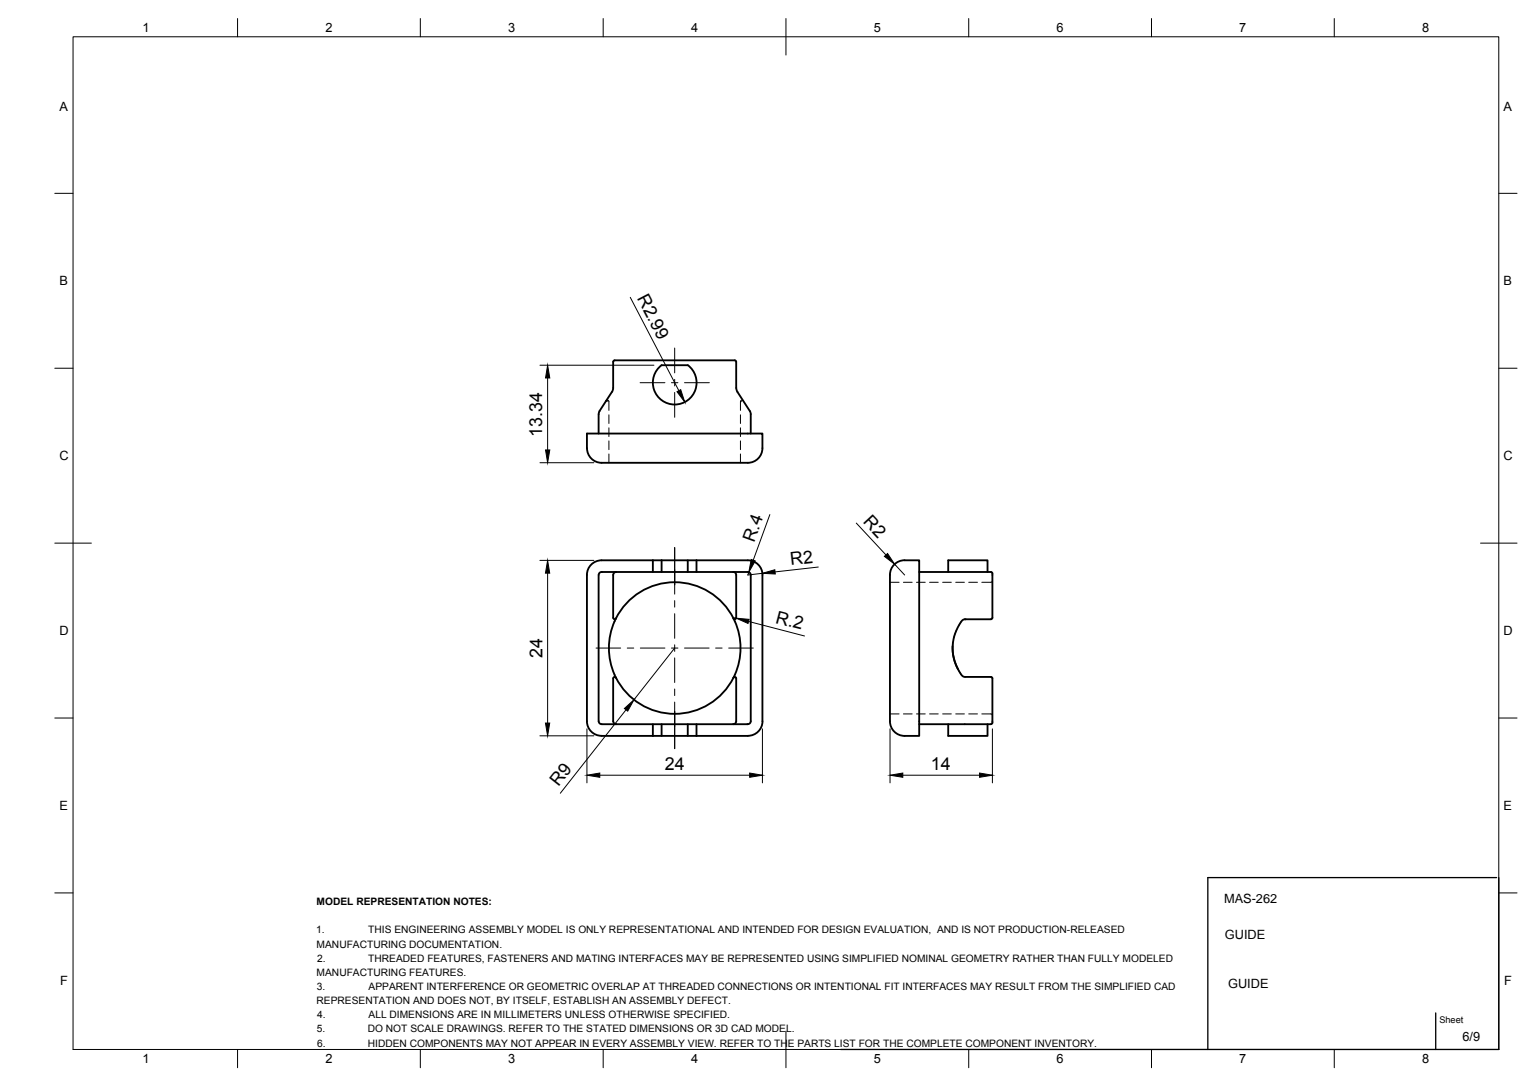
ISO-10303-21;
HEADER;
/* Generated by software containing ST-Developer
 * from STEP Tools, Inc. (www.steptools.com) 
 */

FILE_DESCRIPTION(
/* description */ (''),
/* implementation_level */ '2;1');

FILE_NAME(
/* name */ 'GUIDE.step',
/* time_stamp */ '2026-10-07T02:13:48+06:00',
/* author */ (''),
/* organization */ (''),
/* preprocessor_version */ 'ST-DEVELOPER v20.2',
/* originating_system */ 'Autodesk Translation Framework v15.15.0.0',
/* authorisation */ '');

FILE_SCHEMA (('AUTOMOTIVE_DESIGN { 1 0 10303 214 3 1 1 }'));
ENDSEC;

DATA;
#10=MECHANICAL_DESIGN_GEOMETRIC_PRESENTATION_REPRESENTATION('',(#117),#17042);
#70=B_SPLINE_SURFACE_WITH_KNOTS('',3,3,((#13032,#13033,#13034,#13035,#13036),
(#13037,#13038,#13039,#13040,#13041),(#13042,#13043,#13044,#13045,#13046),
(#13047,#13048,#13049,#13050,#13051),(#13052,#13053,#13054,#13055,#13056),
(#13057,#13058,#13059,#13060,#13061),(#13062,#13063,#13064,#13065,#13066)),
 .UNSPECIFIED.,.F.,.F.,.F.,(4,1,1,1,4),(4,1,4),(0.,0.285714285714286,0.571428571428571,
0.857142857142857,1.),(0.,0.020779022277979,0.0415580445559579),
 .UNSPECIFIED.);
#71=B_SPLINE_SURFACE_WITH_KNOTS('',3,3,((#13080,#13081,#13082,#13083,#13084,
#13085),(#13086,#13087,#13088,#13089,#13090,#13091),(#13092,#13093,#13094,
#13095,#13096,#13097),(#13098,#13099,#13100,#13101,#13102,#13103),(#13104,
#13105,#13106,#13107,#13108,#13109),(#13110,#13111,#13112,#13113,#13114,
#13115),(#13116,#13117,#13118,#13119,#13120,#13121)),.UNSPECIFIED.,.F.,
 .F.,.F.,(4,1,1,1,4),(4,1,1,4),(0.,0.285714285714286,0.571428571428571,
0.857142857142857,1.),(-0.417579612421967,-0.0596542303459957,0.178962691037985,
0.417579612421966),.UNSPECIFIED.);
#72=B_SPLINE_SURFACE_WITH_KNOTS('',3,3,((#13127,#13128,#13129,#13130,#13131),
(#13132,#13133,#13134,#13135,#13136),(#13137,#13138,#13139,#13140,#13141),
(#13142,#13143,#13144,#13145,#13146),(#13147,#13148,#13149,#13150,#13151),
(#13152,#13153,#13154,#13155,#13156),(#13157,#13158,#13159,#13160,#13161)),
 .UNSPECIFIED.,.F.,.F.,.F.,(4,1,1,1,4),(4,1,4),(0.,0.285714285714286,0.571428571428571,
0.857142857142857,1.),(0.,0.0207805027277528,0.0415610054555056),
 .UNSPECIFIED.);
#73=B_SPLINE_SURFACE_WITH_KNOTS('',3,3,((#13236,#13237,#13238,#13239,#13240),
(#13241,#13242,#13243,#13244,#13245),(#13246,#13247,#13248,#13249,#13250),
(#13251,#13252,#13253,#13254,#13255),(#13256,#13257,#13258,#13259,#13260),
(#13261,#13262,#13263,#13264,#13265),(#13266,#13267,#13268,#13269,#13270)),
 .UNSPECIFIED.,.F.,.F.,.F.,(4,1,1,1,4),(4,1,4),(0.,0.285714285714286,0.571428571428571,
0.857142857142857,1.),(0.,0.0207790222779789,0.0415580445559579),
 .UNSPECIFIED.);
#74=B_SPLINE_SURFACE_WITH_KNOTS('',3,3,((#13284,#13285,#13286,#13287,#13288,
#13289),(#13290,#13291,#13292,#13293,#13294,#13295),(#13296,#13297,#13298,
#13299,#13300,#13301),(#13302,#13303,#13304,#13305,#13306,#13307),(#13308,
#13309,#13310,#13311,#13312,#13313),(#13314,#13315,#13316,#13317,#13318,
#13319),(#13320,#13321,#13322,#13323,#13324,#13325)),.UNSPECIFIED.,.F.,
 .F.,.F.,(4,1,1,1,4),(4,1,1,4),(0.,0.285714285714286,0.571428571428571,
0.857142857142857,1.),(-0.417579612421968,-0.0596542303459959,0.178962691037985,
0.417579612421966),.UNSPECIFIED.);
#75=B_SPLINE_SURFACE_WITH_KNOTS('',3,3,((#13331,#13332,#13333,#13334,#13335),
(#13336,#13337,#13338,#13339,#13340),(#13341,#13342,#13343,#13344,#13345),
(#13346,#13347,#13348,#13349,#13350),(#13351,#13352,#13353,#13354,#13355),
(#13356,#13357,#13358,#13359,#13360),(#13361,#13362,#13363,#13364,#13365)),
 .UNSPECIFIED.,.F.,.F.,.F.,(4,1,1,1,4),(4,1,4),(0.,0.285714285714286,0.571428571428571,
0.857142857142857,1.),(0.,0.0207805027277526,0.0415610054555052),
 .UNSPECIFIED.);
#93=SHAPE_REPRESENTATION_RELATIONSHIP('SRR','None',#17089,#105);
#105=ADVANCED_BREP_SHAPE_REPRESENTATION('',(#129),#17033);
#117=STYLED_ITEM('',(#17154),#129);
#129=MANIFOLD_SOLID_BREP('Body1',#8118);
#158=FACE_BOUND('',#1181,.T.);
#159=FACE_BOUND('',#1228,.T.);
#160=FACE_BOUND('',#1237,.T.);
#161=FACE_BOUND('',#1260,.T.);
#188=(
BOUNDED_SURFACE()
B_SPLINE_SURFACE(2,2,((#13423,#13424,#13425),(#13426,#13427,#13428),(#13429,
#13430,#13431)),.UNSPECIFIED.,.F.,.F.,.F.)
B_SPLINE_SURFACE_WITH_KNOTS((3,3),(3,3),(-1.5707963267949,1.77635683940025E-13),
(0.,1.5707963267949),.UNSPECIFIED.)
GEOMETRIC_REPRESENTATION_ITEM()
RATIONAL_B_SPLINE_SURFACE(((1.,0.707106781186548,1.),(0.707106781186393,
0.499999999999891,0.707106781186393),(1.,0.707106781186548,1.)))
REPRESENTATION_ITEM('')
SURFACE()
);
#189=(
BOUNDED_SURFACE()
B_SPLINE_SURFACE(2,2,((#13443,#13444,#13445),(#13446,#13447,#13448),(#13449,
#13450,#13451)),.UNSPECIFIED.,.F.,.F.,.F.)
B_SPLINE_SURFACE_WITH_KNOTS((3,3),(3,3),(-1.5707963267949,0.),(-1.5707963267949,
5.55111512312578E-15),.UNSPECIFIED.)
GEOMETRIC_REPRESENTATION_ITEM()
RATIONAL_B_SPLINE_SURFACE(((1.,0.707106781186546,1.),(0.707106781186793,
0.500000000000172,0.707106781186793),(1.,0.707106781186546,1.)))
REPRESENTATION_ITEM('')
SURFACE()
);
#190=(
BOUNDED_SURFACE()
B_SPLINE_SURFACE(2,2,((#13465,#13466,#13467),(#13468,#13469,#13470),(#13471,
#13472,#13473)),.UNSPECIFIED.,.F.,.F.,.F.)
B_SPLINE_SURFACE_WITH_KNOTS((3,3),(3,3),(-1.5707963267949,0.),(-3.14159265358979,
-1.5707963267949),.UNSPECIFIED.)
GEOMETRIC_REPRESENTATION_ITEM()
RATIONAL_B_SPLINE_SURFACE(((1.,0.707106781186548,1.),(0.707106781186801,
0.50000000000018,0.707106781186801),(1.,0.707106781186548,1.)))
REPRESENTATION_ITEM('')
SURFACE()
);
#191=(
BOUNDED_SURFACE()
B_SPLINE_SURFACE(2,2,((#13485,#13486,#13487),(#13488,#13489,#13490),(#13491,
#13492,#13493)),.UNSPECIFIED.,.F.,.F.,.F.)
B_SPLINE_SURFACE_WITH_KNOTS((3,3),(3,3),(-1.5707963267949,0.),(1.5707963267949,
3.14159265358979),.UNSPECIFIED.)
GEOMETRIC_REPRESENTATION_ITEM()
RATIONAL_B_SPLINE_SURFACE(((1.,0.707106781186547,1.),(0.707106781186801,
0.500000000000179,0.707106781186801),(1.,0.707106781186547,1.)))
REPRESENTATION_ITEM('')
SURFACE()
);
#192=(
BOUNDED_SURFACE()
B_SPLINE_SURFACE(2,2,((#13513,#13514,#13515),(#13516,#13517,#13518),(#13519,
#13520,#13521)),.UNSPECIFIED.,.F.,.F.,.F.)
B_SPLINE_SURFACE_WITH_KNOTS((3,3),(3,3),(-8.32667268468867E-15,1.57079632679493),
(-1.57079632679491,-0.994301061223377),.UNSPECIFIED.)
GEOMETRIC_REPRESENTATION_ITEM()
RATIONAL_B_SPLINE_SURFACE(((1.,0.958743497277462,1.),(0.707106781186526,
0.677934028343379,0.707106781186526),(1.,0.958743497277462,1.)))
REPRESENTATION_ITEM('')
SURFACE()
);
#193=(
BOUNDED_SURFACE()
B_SPLINE_SURFACE(2,2,((#13547,#13548,#13549),(#13550,#13551,#13552),(#13553,
#13554,#13555)),.UNSPECIFIED.,.F.,.F.,.F.)
B_SPLINE_SURFACE_WITH_KNOTS((3,3),(3,3),(0.,1.57079632679491),(0.994301061223376,
1.5707963267949),.UNSPECIFIED.)
GEOMETRIC_REPRESENTATION_ITEM()
RATIONAL_B_SPLINE_SURFACE(((1.,0.958743497277463,1.),(0.707106781186533,
0.677934028343387,0.707106781186533),(1.,0.958743497277463,1.)))
REPRESENTATION_ITEM('')
SURFACE()
);
#194=(
BOUNDED_SURFACE()
B_SPLINE_SURFACE(2,2,((#13571,#13572,#13573),(#13574,#13575,#13576),(#13577,
#13578,#13579)),.UNSPECIFIED.,.F.,.F.,.F.)
B_SPLINE_SURFACE_WITH_KNOTS((3,3),(3,3),(0.,1.57079632679492),(1.5707963267949,
2.14729159236641),.UNSPECIFIED.)
GEOMETRIC_REPRESENTATION_ITEM()
RATIONAL_B_SPLINE_SURFACE(((1.,0.958743497277464,1.),(0.707106781186532,
0.677934028343386,0.707106781186532),(1.,0.958743497277464,1.)))
REPRESENTATION_ITEM('')
SURFACE()
);
#195=(
BOUNDED_SURFACE()
B_SPLINE_SURFACE(2,2,((#13605,#13606,#13607),(#13608,#13609,#13610),(#13611,
#13612,#13613)),.UNSPECIFIED.,.F.,.F.,.F.)
B_SPLINE_SURFACE_WITH_KNOTS((3,3),(3,3),(0.,1.57079632679492),(-2.14729159236642,
-1.57079632679489),.UNSPECIFIED.)
GEOMETRIC_REPRESENTATION_ITEM()
RATIONAL_B_SPLINE_SURFACE(((1.,0.958743497277463,1.),(0.707106781186532,
0.677934028343385,0.707106781186532),(1.,0.958743497277463,1.)))
REPRESENTATION_ITEM('')
SURFACE()
);
#202=SPHERICAL_SURFACE('',#8655,2.);
#203=SPHERICAL_SURFACE('',#8660,2.);
#204=SPHERICAL_SURFACE('',#8665,2.);
#205=SPHERICAL_SURFACE('',#8667,2.);
#206=SPHERICAL_SURFACE('',#8677,0.2);
#207=SPHERICAL_SURFACE('',#8690,0.2);
#208=SPHERICAL_SURFACE('',#8707,0.2);
#209=SPHERICAL_SURFACE('',#8720,0.2);
#220=TOROIDAL_SURFACE('',#8702,9.2,0.2);
#221=TOROIDAL_SURFACE('',#8731,9.2,0.2);
#222=TOROIDAL_SURFACE('',#8762,1.39999999999987,0.4);
#223=TOROIDAL_SURFACE('',#8773,1.39999999999987,0.4);
#224=TOROIDAL_SURFACE('',#8782,1.39999999999987,0.4);
#225=TOROIDAL_SURFACE('',#8793,1.39999999999987,0.4);
#240=ELLIPSE('',#8685,16.7697982864697,9.);
#241=ELLIPSE('',#8686,16.8779777985659,9.2);
#242=ELLIPSE('',#8715,16.7697982864697,9.);
#243=ELLIPSE('',#8716,16.8779777985659,9.2);
#370=PLANE('',#8671);
#371=PLANE('',#8674);
#372=PLANE('',#8675);
#373=PLANE('',#8693);
#374=PLANE('',#8696);
#375=PLANE('',#8699);
#376=PLANE('',#8722);
#377=PLANE('',#8725);
#378=PLANE('',#8728);
#379=PLANE('',#8746);
#380=PLANE('',#8758);
#381=PLANE('',#8769);
#382=PLANE('',#8789);
#383=PLANE('',#8801);
#384=PLANE('',#8802);
#385=PLANE('',#8805);
#386=PLANE('',#8806);
#387=PLANE('',#8807);
#388=PLANE('',#8808);
#389=PLANE('',#8821);
#390=PLANE('',#8824);
#391=PLANE('',#8825);
#671=FACE_OUTER_BOUND('',#1168,.T.);
#672=FACE_OUTER_BOUND('',#1169,.T.);
#673=FACE_OUTER_BOUND('',#1170,.T.);
#674=FACE_OUTER_BOUND('',#1171,.T.);
#675=FACE_OUTER_BOUND('',#1172,.T.);
#676=FACE_OUTER_BOUND('',#1173,.T.);
#677=FACE_OUTER_BOUND('',#1174,.T.);
#678=FACE_OUTER_BOUND('',#1175,.T.);
#679=FACE_OUTER_BOUND('',#1176,.T.);
#680=FACE_OUTER_BOUND('',#1177,.T.);
#681=FACE_OUTER_BOUND('',#1178,.T.);
#682=FACE_OUTER_BOUND('',#1179,.T.);
#683=FACE_OUTER_BOUND('',#1180,.T.);
#684=FACE_OUTER_BOUND('',#1182,.T.);
#685=FACE_OUTER_BOUND('',#1183,.T.);
#686=FACE_OUTER_BOUND('',#1184,.T.);
#687=FACE_OUTER_BOUND('',#1185,.T.);
#688=FACE_OUTER_BOUND('',#1186,.T.);
#689=FACE_OUTER_BOUND('',#1187,.T.);
#690=FACE_OUTER_BOUND('',#1188,.T.);
#691=FACE_OUTER_BOUND('',#1189,.T.);
#692=FACE_OUTER_BOUND('',#1190,.T.);
#693=FACE_OUTER_BOUND('',#1191,.T.);
#694=FACE_OUTER_BOUND('',#1192,.T.);
#695=FACE_OUTER_BOUND('',#1193,.T.);
#696=FACE_OUTER_BOUND('',#1194,.T.);
#697=FACE_OUTER_BOUND('',#1195,.T.);
#698=FACE_OUTER_BOUND('',#1196,.T.);
#699=FACE_OUTER_BOUND('',#1197,.T.);
#700=FACE_OUTER_BOUND('',#1198,.T.);
#701=FACE_OUTER_BOUND('',#1199,.T.);
#702=FACE_OUTER_BOUND('',#1200,.T.);
#703=FACE_OUTER_BOUND('',#1201,.T.);
#704=FACE_OUTER_BOUND('',#1202,.T.);
#705=FACE_OUTER_BOUND('',#1203,.T.);
#706=FACE_OUTER_BOUND('',#1204,.T.);
#707=FACE_OUTER_BOUND('',#1205,.T.);
#708=FACE_OUTER_BOUND('',#1206,.T.);
#709=FACE_OUTER_BOUND('',#1207,.T.);
#710=FACE_OUTER_BOUND('',#1208,.T.);
#711=FACE_OUTER_BOUND('',#1209,.T.);
#712=FACE_OUTER_BOUND('',#1210,.T.);
#713=FACE_OUTER_BOUND('',#1211,.T.);
#714=FACE_OUTER_BOUND('',#1212,.T.);
#715=FACE_OUTER_BOUND('',#1213,.T.);
#716=FACE_OUTER_BOUND('',#1214,.T.);
#717=FACE_OUTER_BOUND('',#1215,.T.);
#718=FACE_OUTER_BOUND('',#1216,.T.);
#719=FACE_OUTER_BOUND('',#1217,.T.);
#720=FACE_OUTER_BOUND('',#1218,.T.);
#721=FACE_OUTER_BOUND('',#1219,.T.);
#722=FACE_OUTER_BOUND('',#1220,.T.);
#723=FACE_OUTER_BOUND('',#1221,.T.);
#724=FACE_OUTER_BOUND('',#1222,.T.);
#725=FACE_OUTER_BOUND('',#1223,.T.);
#726=FACE_OUTER_BOUND('',#1224,.T.);
#727=FACE_OUTER_BOUND('',#1225,.T.);
#728=FACE_OUTER_BOUND('',#1226,.T.);
#729=FACE_OUTER_BOUND('',#1227,.T.);
#730=FACE_OUTER_BOUND('',#1229,.T.);
#731=FACE_OUTER_BOUND('',#1230,.T.);
#732=FACE_OUTER_BOUND('',#1231,.T.);
#733=FACE_OUTER_BOUND('',#1232,.T.);
#734=FACE_OUTER_BOUND('',#1233,.T.);
#735=FACE_OUTER_BOUND('',#1234,.T.);
#736=FACE_OUTER_BOUND('',#1235,.T.);
#737=FACE_OUTER_BOUND('',#1236,.T.);
#738=FACE_OUTER_BOUND('',#1238,.T.);
#739=FACE_OUTER_BOUND('',#1239,.T.);
#740=FACE_OUTER_BOUND('',#1240,.T.);
#741=FACE_OUTER_BOUND('',#1241,.T.);
#742=FACE_OUTER_BOUND('',#1242,.T.);
#743=FACE_OUTER_BOUND('',#1243,.T.);
#744=FACE_OUTER_BOUND('',#1244,.T.);
#745=FACE_OUTER_BOUND('',#1245,.T.);
#746=FACE_OUTER_BOUND('',#1246,.T.);
#747=FACE_OUTER_BOUND('',#1247,.T.);
#748=FACE_OUTER_BOUND('',#1248,.T.);
#749=FACE_OUTER_BOUND('',#1249,.T.);
#750=FACE_OUTER_BOUND('',#1250,.T.);
#751=FACE_OUTER_BOUND('',#1251,.T.);
#752=FACE_OUTER_BOUND('',#1252,.T.);
#753=FACE_OUTER_BOUND('',#1253,.T.);
#754=FACE_OUTER_BOUND('',#1254,.T.);
#755=FACE_OUTER_BOUND('',#1255,.T.);
#756=FACE_OUTER_BOUND('',#1256,.T.);
#757=FACE_OUTER_BOUND('',#1257,.T.);
#758=FACE_OUTER_BOUND('',#1258,.T.);
#759=FACE_OUTER_BOUND('',#1259,.T.);
#1168=EDGE_LOOP('',(#6121,#6122,#6123,#6124));
#1169=EDGE_LOOP('',(#6125,#6126,#6127,#6128));
#1170=EDGE_LOOP('',(#6129,#6130,#6131));
#1171=EDGE_LOOP('',(#6132,#6133,#6134,#6135));
#1172=EDGE_LOOP('',(#6136,#6137,#6138));
#1173=EDGE_LOOP('',(#6139,#6140,#6141,#6142));
#1174=EDGE_LOOP('',(#6143,#6144,#6145));
#1175=EDGE_LOOP('',(#6146,#6147,#6148));
#1176=EDGE_LOOP('',(#6149,#6150,#6151,#6152));
#1177=EDGE_LOOP('',(#6153,#6154,#6155,#6156));
#1178=EDGE_LOOP('',(#6157,#6158,#6159,#6160));
#1179=EDGE_LOOP('',(#6161,#6162,#6163,#6164));
#1180=EDGE_LOOP('',(#6165,#6166,#6167,#6168));
#1181=EDGE_LOOP('',(#6169));
#1182=EDGE_LOOP('',(#6170,#6171,#6172));
#1183=EDGE_LOOP('',(#6173,#6174,#6175,#6176));
#1184=EDGE_LOOP('',(#6177,#6178,#6179,#6180));
#1185=EDGE_LOOP('',(#6181,#6182,#6183,#6184));
#1186=EDGE_LOOP('',(#6185,#6186,#6187,#6188));
#1187=EDGE_LOOP('',(#6189,#6190,#6191,#6192));
#1188=EDGE_LOOP('',(#6193,#6194,#6195));
#1189=EDGE_LOOP('',(#6196,#6197,#6198,#6199));
#1190=EDGE_LOOP('',(#6200,#6201,#6202,#6203));
#1191=EDGE_LOOP('',(#6204,#6205,#6206,#6207,#6208,#6209));
#1192=EDGE_LOOP('',(#6210,#6211,#6212,#6213));
#1193=EDGE_LOOP('',(#6214,#6215,#6216,#6217));
#1194=EDGE_LOOP('',(#6218,#6219,#6220,#6221));
#1195=EDGE_LOOP('',(#6222,#6223,#6224,#6225,#6226));
#1196=EDGE_LOOP('',(#6227,#6228,#6229));
#1197=EDGE_LOOP('',(#6230,#6231,#6232,#6233));
#1198=EDGE_LOOP('',(#6234,#6235,#6236,#6237));
#1199=EDGE_LOOP('',(#6238,#6239,#6240,#6241));
#1200=EDGE_LOOP('',(#6242,#6243,#6244,#6245));
#1201=EDGE_LOOP('',(#6246,#6247,#6248,#6249));
#1202=EDGE_LOOP('',(#6250,#6251,#6252));
#1203=EDGE_LOOP('',(#6253,#6254,#6255,#6256));
#1204=EDGE_LOOP('',(#6257,#6258,#6259,#6260));
#1205=EDGE_LOOP('',(#6261,#6262,#6263,#6264,#6265,#6266));
#1206=EDGE_LOOP('',(#6267,#6268,#6269,#6270));
#1207=EDGE_LOOP('',(#6271,#6272,#6273,#6274));
#1208=EDGE_LOOP('',(#6275,#6276,#6277,#6278));
#1209=EDGE_LOOP('',(#6279,#6280,#6281,#6282));
#1210=EDGE_LOOP('',(#6283,#6284,#6285,#6286));
#1211=EDGE_LOOP('',(#6287,#6288,#6289,#6290));
#1212=EDGE_LOOP('',(#6291,#6292,#6293,#6294));
#1213=EDGE_LOOP('',(#6295,#6296,#6297,#6298));
#1214=EDGE_LOOP('',(#6299,#6300,#6301,#6302));
#1215=EDGE_LOOP('',(#6303,#6304,#6305,#6306,#6307,#6308,#6309,#6310,#6311,
#6312,#6313,#6314,#6315,#6316,#6317,#6318));
#1216=EDGE_LOOP('',(#6319,#6320,#6321,#6322,#6323,#6324));
#1217=EDGE_LOOP('',(#6325,#6326,#6327,#6328));
#1218=EDGE_LOOP('',(#6329,#6330,#6331,#6332));
#1219=EDGE_LOOP('',(#6333,#6334,#6335,#6336));
#1220=EDGE_LOOP('',(#6337,#6338,#6339,#6340));
#1221=EDGE_LOOP('',(#6341,#6342,#6343,#6344));
#1222=EDGE_LOOP('',(#6345,#6346,#6347,#6348,#6349,#6350));
#1223=EDGE_LOOP('',(#6351,#6352,#6353,#6354));
#1224=EDGE_LOOP('',(#6355,#6356,#6357,#6358));
#1225=EDGE_LOOP('',(#6359,#6360,#6361,#6362));
#1226=EDGE_LOOP('',(#6363,#6364,#6365,#6366));
#1227=EDGE_LOOP('',(#6367,#6368,#6369,#6370,#6371,#6372,#6373,#6374,#6375,
#6376,#6377,#6378));
#1228=EDGE_LOOP('',(#6379,#6380));
#1229=EDGE_LOOP('',(#6381,#6382,#6383,#6384));
#1230=EDGE_LOOP('',(#6385,#6386,#6387,#6388));
#1231=EDGE_LOOP('',(#6389,#6390,#6391,#6392));
#1232=EDGE_LOOP('',(#6393,#6394,#6395,#6396));
#1233=EDGE_LOOP('',(#6397,#6398,#6399,#6400));
#1234=EDGE_LOOP('',(#6401,#6402,#6403,#6404));
#1235=EDGE_LOOP('',(#6405,#6406,#6407,#6408));
#1236=EDGE_LOOP('',(#6409,#6410,#6411,#6412,#6413,#6414,#6415,#6416,#6417,
#6418,#6419,#6420));
#1237=EDGE_LOOP('',(#6421,#6422));
#1238=EDGE_LOOP('',(#6423,#6424,#6425,#6426));
#1239=EDGE_LOOP('',(#6427,#6428,#6429,#6430));
#1240=EDGE_LOOP('',(#6431,#6432,#6433,#6434));
#1241=EDGE_LOOP('',(#6435,#6436,#6437,#6438));
#1242=EDGE_LOOP('',(#6439,#6440,#6441,#6442));
#1243=EDGE_LOOP('',(#6443,#6444,#6445,#6446));
#1244=EDGE_LOOP('',(#6447,#6448,#6449,#6450));
#1245=EDGE_LOOP('',(#6451,#6452,#6453,#6454));
#1246=EDGE_LOOP('',(#6455,#6456,#6457,#6458));
#1247=EDGE_LOOP('',(#6459,#6460));
#1248=EDGE_LOOP('',(#6461,#6462,#6463,#6464));
#1249=EDGE_LOOP('',(#6465,#6466));
#1250=EDGE_LOOP('',(#6467,#6468,#6469,#6470));
#1251=EDGE_LOOP('',(#6471,#6472,#6473,#6474));
#1252=EDGE_LOOP('',(#6475,#6476,#6477,#6478));
#1253=EDGE_LOOP('',(#6479,#6480,#6481,#6482));
#1254=EDGE_LOOP('',(#6483,#6484,#6485,#6486));
#1255=EDGE_LOOP('',(#6487,#6488,#6489,#6490));
#1256=EDGE_LOOP('',(#6491,#6492,#6493,#6494));
#1257=EDGE_LOOP('',(#6495,#6496,#6497,#6498));
#1258=EDGE_LOOP('',(#6499,#6500,#6501,#6502));
#1259=EDGE_LOOP('',(#6503,#6504,#6505,#6506,#6507,#6508,#6509,#6510));
#1260=EDGE_LOOP('',(#6511,#6512,#6513,#6514,#6515,#6516,#6517,#6518));
#1666=CIRCLE('',#8650,1.99999999999996);
#1667=CIRCLE('',#8651,2.);
#1668=CIRCLE('',#8653,1.99999999999996);
#1669=CIRCLE('',#8654,2.);
#1670=CIRCLE('',#8656,2.);
#1671=CIRCLE('',#8658,1.99999999999996);
#1672=CIRCLE('',#8659,2.);
#1673=CIRCLE('',#8661,2.);
#1674=CIRCLE('',#8663,1.99999999999996);
#1675=CIRCLE('',#8664,2.);
#1676=CIRCLE('',#8666,2.);
#1677=CIRCLE('',#8668,2.00000000000001);
#1678=CIRCLE('',#8670,2.);
#1679=CIRCLE('',#8673,2.00000000000001);
#1680=CIRCLE('',#8676,9.);
#1681=CIRCLE('',#8678,0.200000000000002);
#1682=CIRCLE('',#8679,0.2);
#1683=CIRCLE('',#8680,0.200000000000002);
#1684=CIRCLE('',#8682,0.200000000000008);
#1685=CIRCLE('',#8683,0.199999999999995);
#1686=CIRCLE('',#8684,0.199999999999991);
#1687=CIRCLE('',#8687,0.2);
#1688=CIRCLE('',#8689,0.200000000000012);
#1689=CIRCLE('',#8691,0.200000000000002);
#1690=CIRCLE('',#8692,0.2);
#1691=CIRCLE('',#8695,0.999999999999871);
#1692=CIRCLE('',#8698,0.999999999999871);
#1693=CIRCLE('',#8701,0.2);
#1694=CIRCLE('',#8703,9.);
#1695=CIRCLE('',#8704,9.);
#1696=CIRCLE('',#8705,0.2);
#1697=CIRCLE('',#8706,9.2);
#1698=CIRCLE('',#8708,0.199999999999995);
#1699=CIRCLE('',#8709,0.2);
#1700=CIRCLE('',#8710,0.199999999999995);
#1701=CIRCLE('',#8712,0.200000000000009);
#1702=CIRCLE('',#8713,0.199999999999999);
#1703=CIRCLE('',#8714,0.199999999999995);
#1704=CIRCLE('',#8717,0.2);
#1705=CIRCLE('',#8719,0.200000000000012);
#1706=CIRCLE('',#8721,0.199999999999995);
#1707=CIRCLE('',#8724,0.999999999999871);
#1708=CIRCLE('',#8727,0.999999999999871);
#1709=CIRCLE('',#8730,0.2);
#1710=CIRCLE('',#8732,9.2);
#1711=CIRCLE('',#8733,9.);
#1712=CIRCLE('',#8735,0.2);
#1713=CIRCLE('',#8736,0.2);
#1714=CIRCLE('',#8737,0.2);
#1715=CIRCLE('',#8738,0.4);
#1716=CIRCLE('',#8740,0.2);
#1717=CIRCLE('',#8741,0.2);
#1718=CIRCLE('',#8742,0.4);
#1719=CIRCLE('',#8744,0.4);
#1720=CIRCLE('',#8748,0.2);
#1721=CIRCLE('',#8749,0.2);
#1722=CIRCLE('',#8750,0.2);
#1723=CIRCLE('',#8751,0.4);
#1724=CIRCLE('',#8753,0.2);
#1725=CIRCLE('',#8754,0.2);
#1726=CIRCLE('',#8755,0.4);
#1727=CIRCLE('',#8757,0.4);
#1728=CIRCLE('',#8760,0.4);
#1729=CIRCLE('',#8761,0.399999999999992);
#1730=CIRCLE('',#8763,0.4);
#1731=CIRCLE('',#8764,1.39999999999987);
#1732=CIRCLE('',#8766,0.4);
#1733=CIRCLE('',#8767,0.800000000000059);
#1734=CIRCLE('',#8768,0.400000000000058);
#1735=CIRCLE('',#8770,1.39999999999987);
#1736=CIRCLE('',#8771,0.400000000000058);
#1737=CIRCLE('',#8772,2.98575787723652);
#1738=CIRCLE('',#8774,0.400000000000004);
#1739=CIRCLE('',#8776,0.399999999999992);
#1740=CIRCLE('',#8777,0.399999999999994);
#1741=CIRCLE('',#8778,0.800000000000059);
#1742=CIRCLE('',#8780,0.4);
#1743=CIRCLE('',#8781,0.399999999999991);
#1744=CIRCLE('',#8783,0.4);
#1745=CIRCLE('',#8784,1.39999999999987);
#1746=CIRCLE('',#8786,0.4);
#1747=CIRCLE('',#8787,0.800000000000059);
#1748=CIRCLE('',#8788,0.400000000000058);
#1749=CIRCLE('',#8790,1.39999999999987);
#1750=CIRCLE('',#8791,0.400000000000058);
#1751=CIRCLE('',#8792,2.98575787723652);
#1752=CIRCLE('',#8794,0.400000000000005);
#1753=CIRCLE('',#8796,0.399999999999992);
#1754=CIRCLE('',#8797,0.399999999999994);
#1755=CIRCLE('',#8798,0.800000000000059);
#1756=CIRCLE('',#8804,2.98575787723652);
#1757=CIRCLE('',#8809,2.98575787723652);
#1758=CIRCLE('',#8812,0.399999999999998);
#1759=CIRCLE('',#8814,0.4);
#1760=CIRCLE('',#8816,0.400000000000004);
#1761=CIRCLE('',#8818,0.4);
#1762=CIRCLE('',#8820,2.);
#1763=CIRCLE('',#8823,2.);
#1952=B_SPLINE_CURVE_WITH_KNOTS('',3,(#13070,#13071,#13072,#13073,#13074),
 .UNSPECIFIED.,.F.,.F.,(4,1,4),(-0.0415580445559579,-0.020779022277979,
0.),.UNSPECIFIED.);
#1953=B_SPLINE_CURVE_WITH_KNOTS('',3,(#13075,#13076,#13077,#13078,#13079),
 .UNSPECIFIED.,.F.,.F.,(4,1,4),(0.,0.020779022277979,0.0415580445559579),
 .UNSPECIFIED.);
#1954=B_SPLINE_CURVE_WITH_KNOTS('',3,(#13165,#13166,#13167,#13168,#13169),
 .UNSPECIFIED.,.F.,.F.,(4,1,4),(-0.0415610054555056,-0.0207805027277528,
0.),.UNSPECIFIED.);
#1955=B_SPLINE_CURVE_WITH_KNOTS('',3,(#13170,#13171,#13172,#13173,#13174),
 .UNSPECIFIED.,.F.,.F.,(4,1,4),(0.,0.0207805027277528,0.0415610054555056),
 .UNSPECIFIED.);
#1956=B_SPLINE_CURVE_WITH_KNOTS('',3,(#13274,#13275,#13276,#13277,#13278),
 .UNSPECIFIED.,.F.,.F.,(4,1,4),(-0.0415580445559579,-0.0207790222779789,
0.),.UNSPECIFIED.);
#1957=B_SPLINE_CURVE_WITH_KNOTS('',3,(#13279,#13280,#13281,#13282,#13283),
 .UNSPECIFIED.,.F.,.F.,(4,1,4),(0.,0.0207790222779789,0.0415580445559579),
 .UNSPECIFIED.);
#1958=B_SPLINE_CURVE_WITH_KNOTS('',3,(#13369,#13370,#13371,#13372,#13373),
 .UNSPECIFIED.,.F.,.F.,(4,1,4),(-0.0415610054555052,-0.0207805027277526,
0.),.UNSPECIFIED.);
#1959=B_SPLINE_CURVE_WITH_KNOTS('',3,(#13374,#13375,#13376,#13377,#13378),
 .UNSPECIFIED.,.F.,.F.,(4,1,4),(0.,0.0207805027277526,0.0415610054555052),
 .UNSPECIFIED.);
#2337=LINE('',#12963,#2915);
#2338=LINE('',#12966,#2916);
#2339=LINE('',#12971,#2917);
#2340=LINE('',#12974,#2918);
#2341=LINE('',#12981,#2919);
#2342=LINE('',#12984,#2920);
#2343=LINE('',#12991,#2921);
#2344=LINE('',#12993,#2922);
#2345=LINE('',#13000,#2923);
#2346=LINE('',#13003,#2924);
#2347=LINE('',#13006,#2925);
#2348=LINE('',#13007,#2926);
#2349=LINE('',#13010,#2927);
#2350=LINE('',#13014,#2928);
#2351=LINE('',#13015,#2929);
#2352=LINE('',#13030,#2930);
#2353=LINE('',#13031,#2931);
#2354=LINE('',#13179,#2932);
#2355=LINE('',#13180,#2933);
#2356=LINE('',#13187,#2934);
#2357=LINE('',#13189,#2935);
#2358=LINE('',#13190,#2936);
#2359=LINE('',#13193,#2937);
#2360=LINE('',#13197,#2938);
#2361=LINE('',#13199,#2939);
#2362=LINE('',#13201,#2940);
#2363=LINE('',#13202,#2941);
#2364=LINE('',#13205,#2942);
#2365=LINE('',#13209,#2943);
#2366=LINE('',#13210,#2944);
#2367=LINE('',#13213,#2945);
#2368=LINE('',#13234,#2946);
#2369=LINE('',#13235,#2947);
#2370=LINE('',#13382,#2948);
#2371=LINE('',#13383,#2949);
#2372=LINE('',#13388,#2950);
#2373=LINE('',#13390,#2951);
#2374=LINE('',#13391,#2952);
#2375=LINE('',#13394,#2953);
#2376=LINE('',#13398,#2954);
#2377=LINE('',#13400,#2955);
#2378=LINE('',#13402,#2956);
#2379=LINE('',#13403,#2957);
#2380=LINE('',#13406,#2958);
#2381=LINE('',#13410,#2959);
#2382=LINE('',#13411,#2960);
#2383=LINE('',#13414,#2961);
#2384=LINE('',#13422,#2962);
#2385=LINE('',#13441,#2963);
#2386=LINE('',#13442,#2964);
#2387=LINE('',#13457,#2965);
#2388=LINE('',#13459,#2966);
#2389=LINE('',#13464,#2967);
#2390=LINE('',#13483,#2968);
#2391=LINE('',#13484,#2969);
#2392=LINE('',#13499,#2970);
#2393=LINE('',#13506,#2971);
#2394=LINE('',#13512,#2972);
#2395=LINE('',#13531,#2973);
#2396=LINE('',#13535,#2974);
#2397=LINE('',#13537,#2975);
#2398=LINE('',#13538,#2976);
#2399=LINE('',#13542,#2977);
#2400=LINE('',#13564,#2978);
#2401=LINE('',#13570,#2979);
#2402=LINE('',#13589,#2980);
#2403=LINE('',#13593,#2981);
#2404=LINE('',#13595,#2982);
#2405=LINE('',#13596,#2983);
#2406=LINE('',#13599,#2984);
#2407=LINE('',#13618,#2985);
#2408=LINE('',#13620,#2986);
#2409=LINE('',#13623,#2987);
#2410=LINE('',#13625,#2988);
#2411=LINE('',#13626,#2989);
#2412=LINE('',#13629,#2990);
#2413=LINE('',#13631,#2991);
#2414=LINE('',#13632,#2992);
#2415=LINE('',#13635,#2993);
#2416=LINE('',#13638,#2994);
#2417=LINE('',#13640,#2995);
#2418=LINE('',#13644,#2996);
#2419=LINE('',#13646,#2997);
#2420=LINE('',#13647,#2998);
#2421=LINE('',#13661,#2999);
#2422=LINE('',#13665,#3000);
#2423=LINE('',#13666,#3001);
#2424=LINE('',#13669,#3002);
#2425=LINE('',#13672,#3003);
#2915=VECTOR('',#10348,20.);
#2916=VECTOR('',#10351,20.);
#2917=VECTOR('',#10356,20.);
#2918=VECTOR('',#10359,20.);
#2919=VECTOR('',#10368,20.);
#2920=VECTOR('',#10371,20.);
#2921=VECTOR('',#10380,20.);
#2922=VECTOR('',#10383,20.);
#2923=VECTOR('',#10394,20.);
#2924=VECTOR('',#10397,20.);
#2925=VECTOR('',#10400,20.);
#2926=VECTOR('',#10401,20.);
#2927=VECTOR('',#10404,20.);
#2928=VECTOR('',#10409,20.);
#2929=VECTOR('',#10410,20.);
#2930=VECTOR('',#10427,20.);
#2931=VECTOR('',#10428,20.);
#2932=VECTOR('',#10443,20.);
#2933=VECTOR('',#10444,20.);
#2934=VECTOR('',#10453,20.);
#2935=VECTOR('',#10454,20.);
#2936=VECTOR('',#10455,20.);
#2937=VECTOR('',#10458,20.);
#2938=VECTOR('',#10463,20.);
#2939=VECTOR('',#10464,20.);
#2940=VECTOR('',#10465,20.);
#2941=VECTOR('',#10466,20.);
#2942=VECTOR('',#10469,20.);
#2943=VECTOR('',#10474,20.);
#2944=VECTOR('',#10475,20.);
#2945=VECTOR('',#10478,20.);
#2946=VECTOR('',#10503,20.);
#2947=VECTOR('',#10504,20.);
#2948=VECTOR('',#10519,20.);
#2949=VECTOR('',#10520,20.);
#2950=VECTOR('',#10527,20.);
#2951=VECTOR('',#10528,20.);
#2952=VECTOR('',#10529,20.);
#2953=VECTOR('',#10532,20.);
#2954=VECTOR('',#10537,20.);
#2955=VECTOR('',#10538,20.);
#2956=VECTOR('',#10539,20.);
#2957=VECTOR('',#10540,20.);
#2958=VECTOR('',#10543,20.);
#2959=VECTOR('',#10548,20.);
#2960=VECTOR('',#10549,20.);
#2961=VECTOR('',#10552,20.);
#2962=VECTOR('',#10565,20.);
#2963=VECTOR('',#10576,20.);
#2964=VECTOR('',#10577,20.);
#2965=VECTOR('',#10586,20.);
#2966=VECTOR('',#10589,9.);
#2967=VECTOR('',#10596,20.);
#2968=VECTOR('',#10607,20.);
#2969=VECTOR('',#10608,20.);
#2970=VECTOR('',#10617,20.);
#2971=VECTOR('',#10626,20.);
#2972=VECTOR('',#10635,20.);
#2973=VECTOR('',#10646,20.);
#2974=VECTOR('',#10649,20.);
#2975=VECTOR('',#10650,20.);
#2976=VECTOR('',#10651,20.);
#2977=VECTOR('',#10654,20.);
#2978=VECTOR('',#10673,20.);
#2979=VECTOR('',#10682,20.);
#2980=VECTOR('',#10693,20.);
#2981=VECTOR('',#10696,20.);
#2982=VECTOR('',#10697,20.);
#2983=VECTOR('',#10698,20.);
#2984=VECTOR('',#10699,20.);
#2985=VECTOR('',#10716,20.);
#2986=VECTOR('',#10719,20.);
#2987=VECTOR('',#10722,20.);
#2988=VECTOR('',#10723,20.);
#2989=VECTOR('',#10724,20.);
#2990=VECTOR('',#10727,20.);
#2991=VECTOR('',#10728,20.);
#2992=VECTOR('',#10729,20.);
#2993=VECTOR('',#10732,20.);
#2994=VECTOR('',#10735,20.);
#2995=VECTOR('',#10738,20.);
#2996=VECTOR('',#10743,20.);
#2997=VECTOR('',#10744,20.);
#2998=VECTOR('',#10745,20.);
#2999=VECTOR('',#10770,20.);
#3000=VECTOR('',#10775,20.);
#3001=VECTOR('',#10776,20.);
#3002=VECTOR('',#10779,20.);
#3003=VECTOR('',#10784,20.);
#3505=VERTEX_POINT('',#12959);
#3506=VERTEX_POINT('',#12960);
#3507=VERTEX_POINT('',#12962);
#3508=VERTEX_POINT('',#12964);
#3509=VERTEX_POINT('',#12968);
#3510=VERTEX_POINT('',#12970);
#3511=VERTEX_POINT('',#12972);
#3512=VERTEX_POINT('',#12978);
#3513=VERTEX_POINT('',#12980);
#3514=VERTEX_POINT('',#12982);
#3515=VERTEX_POINT('',#12988);
#3516=VERTEX_POINT('',#12990);
#3517=VERTEX_POINT('',#12999);
#3518=VERTEX_POINT('',#13001);
#3519=VERTEX_POINT('',#13005);
#3520=VERTEX_POINT('',#13009);
#3521=VERTEX_POINT('',#13013);
#3522=VERTEX_POINT('',#13017);
#3523=VERTEX_POINT('',#13020);
#3524=VERTEX_POINT('',#13021);
#3525=VERTEX_POINT('',#13023);
#3526=VERTEX_POINT('',#13027);
#3527=VERTEX_POINT('',#13028);
#3528=VERTEX_POINT('',#13067);
#3529=VERTEX_POINT('',#13068);
#3530=VERTEX_POINT('',#13122);
#3531=VERTEX_POINT('',#13123);
#3532=VERTEX_POINT('',#13162);
#3533=VERTEX_POINT('',#13163);
#3534=VERTEX_POINT('',#13176);
#3535=VERTEX_POINT('',#13177);
#3536=VERTEX_POINT('',#13182);
#3537=VERTEX_POINT('',#13186);
#3538=VERTEX_POINT('',#13188);
#3539=VERTEX_POINT('',#13192);
#3540=VERTEX_POINT('',#13196);
#3541=VERTEX_POINT('',#13198);
#3542=VERTEX_POINT('',#13200);
#3543=VERTEX_POINT('',#13204);
#3544=VERTEX_POINT('',#13208);
#3545=VERTEX_POINT('',#13212);
#3546=VERTEX_POINT('',#13216);
#3547=VERTEX_POINT('',#13218);
#3548=VERTEX_POINT('',#13220);
#3549=VERTEX_POINT('',#13224);
#3550=VERTEX_POINT('',#13225);
#3551=VERTEX_POINT('',#13227);
#3552=VERTEX_POINT('',#13231);
#3553=VERTEX_POINT('',#13232);
#3554=VERTEX_POINT('',#13271);
#3555=VERTEX_POINT('',#13272);
#3556=VERTEX_POINT('',#13326);
#3557=VERTEX_POINT('',#13327);
#3558=VERTEX_POINT('',#13366);
#3559=VERTEX_POINT('',#13367);
#3560=VERTEX_POINT('',#13380);
#3561=VERTEX_POINT('',#13387);
#3562=VERTEX_POINT('',#13389);
#3563=VERTEX_POINT('',#13393);
#3564=VERTEX_POINT('',#13397);
#3565=VERTEX_POINT('',#13399);
#3566=VERTEX_POINT('',#13401);
#3567=VERTEX_POINT('',#13405);
#3568=VERTEX_POINT('',#13409);
#3569=VERTEX_POINT('',#13413);
#3570=VERTEX_POINT('',#13420);
#3571=VERTEX_POINT('',#13432);
#3572=VERTEX_POINT('',#13433);
#3573=VERTEX_POINT('',#13438);
#3574=VERTEX_POINT('',#13439);
#3575=VERTEX_POINT('',#13455);
#3576=VERTEX_POINT('',#13462);
#3577=VERTEX_POINT('',#13474);
#3578=VERTEX_POINT('',#13475);
#3579=VERTEX_POINT('',#13480);
#3580=VERTEX_POINT('',#13481);
#3581=VERTEX_POINT('',#13497);
#3582=VERTEX_POINT('',#13502);
#3583=VERTEX_POINT('',#13504);
#3584=VERTEX_POINT('',#13508);
#3585=VERTEX_POINT('',#13522);
#3586=VERTEX_POINT('',#13523);
#3587=VERTEX_POINT('',#13528);
#3588=VERTEX_POINT('',#13530);
#3589=VERTEX_POINT('',#13532);
#3590=VERTEX_POINT('',#13534);
#3591=VERTEX_POINT('',#13536);
#3592=VERTEX_POINT('',#13539);
#3593=VERTEX_POINT('',#13540);
#3594=VERTEX_POINT('',#13556);
#3595=VERTEX_POINT('',#13560);
#3596=VERTEX_POINT('',#13562);
#3597=VERTEX_POINT('',#13566);
#3598=VERTEX_POINT('',#13580);
#3599=VERTEX_POINT('',#13581);
#3600=VERTEX_POINT('',#13586);
#3601=VERTEX_POINT('',#13588);
#3602=VERTEX_POINT('',#13590);
#3603=VERTEX_POINT('',#13592);
#3604=VERTEX_POINT('',#13594);
#3605=VERTEX_POINT('',#13597);
#3606=VERTEX_POINT('',#13598);
#3607=VERTEX_POINT('',#13614);
#3608=VERTEX_POINT('',#13622);
#3609=VERTEX_POINT('',#13624);
#3610=VERTEX_POINT('',#13628);
#3611=VERTEX_POINT('',#13630);
#3612=VERTEX_POINT('',#13634);
#3613=VERTEX_POINT('',#13636);
#3614=VERTEX_POINT('',#13643);
#3615=VERTEX_POINT('',#13645);
#3616=VERTEX_POINT('',#13660);
#3617=VERTEX_POINT('',#13664);
#3618=VERTEX_POINT('',#13668);
#4428=EDGE_CURVE('',#3505,#3506,#1666,.T.);
#4429=EDGE_CURVE('',#3506,#3507,#2337,.T.);
#4430=EDGE_CURVE('',#3507,#3508,#1667,.T.);
#4431=EDGE_CURVE('',#3508,#3505,#2338,.T.);
#4432=EDGE_CURVE('',#3508,#3509,#1668,.T.);
#4433=EDGE_CURVE('',#3509,#3510,#2339,.T.);
#4434=EDGE_CURVE('',#3510,#3511,#1669,.T.);
#4435=EDGE_CURVE('',#3511,#3508,#2340,.T.);
#4436=EDGE_CURVE('',#3507,#3509,#1670,.T.);
#4437=EDGE_CURVE('',#3511,#3512,#1671,.T.);
#4438=EDGE_CURVE('',#3512,#3513,#2341,.T.);
#4439=EDGE_CURVE('',#3513,#3514,#1672,.T.);
#4440=EDGE_CURVE('',#3514,#3511,#2342,.T.);
#4441=EDGE_CURVE('',#3510,#3512,#1673,.T.);
#4442=EDGE_CURVE('',#3514,#3515,#1674,.T.);
#4443=EDGE_CURVE('',#3515,#3516,#2343,.T.);
#4444=EDGE_CURVE('',#3516,#3505,#1675,.T.);
#4445=EDGE_CURVE('',#3505,#3514,#2344,.T.);
#4446=EDGE_CURVE('',#3513,#3515,#1676,.T.);
#4447=EDGE_CURVE('',#3516,#3506,#1677,.T.);
#4448=EDGE_CURVE('',#3517,#3507,#2345,.T.);
#4449=EDGE_CURVE('',#3517,#3518,#1678,.T.);
#4450=EDGE_CURVE('',#3518,#3509,#2346,.T.);
#4451=EDGE_CURVE('',#3519,#3506,#2347,.T.);
#4452=EDGE_CURVE('',#3519,#3517,#2348,.T.);
#4453=EDGE_CURVE('',#3520,#3516,#2349,.T.);
#4454=EDGE_CURVE('',#3520,#3519,#1679,.T.);
#4455=EDGE_CURVE('',#3521,#3515,#2350,.T.);
#4456=EDGE_CURVE('',#3521,#3520,#2351,.T.);
#4457=EDGE_CURVE('',#3522,#3522,#1680,.T.);
#4458=EDGE_CURVE('',#3523,#3524,#1681,.T.);
#4459=EDGE_CURVE('',#3524,#3525,#1682,.T.);
#4460=EDGE_CURVE('',#3525,#3523,#1683,.T.);
#4461=EDGE_CURVE('',#3526,#3527,#1684,.T.);
#4462=EDGE_CURVE('',#3527,#3524,#2352,.T.);
#4463=EDGE_CURVE('',#3523,#3526,#2353,.T.);
#4464=EDGE_CURVE('',#3528,#3529,#1685,.T.);
#4465=EDGE_CURVE('',#3529,#3527,#1952,.T.);
#4466=EDGE_CURVE('',#3526,#3528,#1953,.T.);
#4467=EDGE_CURVE('',#3530,#3531,#1686,.T.);
#4468=EDGE_CURVE('',#3531,#3529,#240,.T.);
#4469=EDGE_CURVE('',#3528,#3530,#241,.T.);
#4470=EDGE_CURVE('',#3532,#3533,#1687,.T.);
#4471=EDGE_CURVE('',#3533,#3531,#1954,.T.);
#4472=EDGE_CURVE('',#3530,#3532,#1955,.T.);
#4473=EDGE_CURVE('',#3534,#3535,#1688,.T.);
#4474=EDGE_CURVE('',#3535,#3533,#2354,.T.);
#4475=EDGE_CURVE('',#3532,#3534,#2355,.T.);
#4476=EDGE_CURVE('',#3534,#3536,#1689,.T.);
#4477=EDGE_CURVE('',#3536,#3535,#1690,.T.);
#4478=EDGE_CURVE('',#3532,#3537,#2356,.T.);
#4479=EDGE_CURVE('',#3538,#3537,#2357,.T.);
#4480=EDGE_CURVE('',#3534,#3538,#2358,.T.);
#4481=EDGE_CURVE('',#3539,#3530,#2359,.T.);
#4482=EDGE_CURVE('',#3537,#3539,#1691,.T.);
#4483=EDGE_CURVE('',#3528,#3540,#2360,.T.);
#4484=EDGE_CURVE('',#3541,#3540,#2361,.T.);
#4485=EDGE_CURVE('',#3541,#3542,#2362,.T.);
#4486=EDGE_CURVE('',#3539,#3542,#2363,.T.);
#4487=EDGE_CURVE('',#3543,#3526,#2364,.T.);
#4488=EDGE_CURVE('',#3540,#3543,#1692,.T.);
#4489=EDGE_CURVE('',#3544,#3523,#2365,.T.);
#4490=EDGE_CURVE('',#3543,#3544,#2366,.T.);
#4491=EDGE_CURVE('',#3525,#3545,#2367,.T.);
#4492=EDGE_CURVE('',#3544,#3545,#1693,.T.);
#4493=EDGE_CURVE('',#3524,#3546,#1694,.T.);
#4494=EDGE_CURVE('',#3546,#3547,#1695,.T.);
#4495=EDGE_CURVE('',#3548,#3547,#1696,.T.);
#4496=EDGE_CURVE('',#3548,#3525,#1697,.T.);
#4497=EDGE_CURVE('',#3549,#3550,#1698,.T.);
#4498=EDGE_CURVE('',#3550,#3551,#1699,.T.);
#4499=EDGE_CURVE('',#3551,#3549,#1700,.T.);
#4500=EDGE_CURVE('',#3552,#3553,#1701,.T.);
#4501=EDGE_CURVE('',#3553,#3550,#2368,.T.);
#4502=EDGE_CURVE('',#3549,#3552,#2369,.T.);
#4503=EDGE_CURVE('',#3554,#3555,#1702,.T.);
#4504=EDGE_CURVE('',#3555,#3553,#1956,.T.);
#4505=EDGE_CURVE('',#3552,#3554,#1957,.T.);
#4506=EDGE_CURVE('',#3556,#3557,#1703,.T.);
#4507=EDGE_CURVE('',#3557,#3555,#242,.T.);
#4508=EDGE_CURVE('',#3554,#3556,#243,.T.);
#4509=EDGE_CURVE('',#3558,#3559,#1704,.T.);
#4510=EDGE_CURVE('',#3559,#3557,#1958,.T.);
#4511=EDGE_CURVE('',#3556,#3558,#1959,.T.);
#4512=EDGE_CURVE('',#3560,#3547,#1705,.T.);
#4513=EDGE_CURVE('',#3547,#3559,#2370,.T.);
#4514=EDGE_CURVE('',#3558,#3560,#2371,.T.);
#4515=EDGE_CURVE('',#3560,#3548,#1706,.T.);
#4516=EDGE_CURVE('',#3561,#3558,#2372,.T.);
#4517=EDGE_CURVE('',#3562,#3561,#2373,.T.);
#4518=EDGE_CURVE('',#3560,#3562,#2374,.T.);
#4519=EDGE_CURVE('',#3563,#3556,#2375,.T.);
#4520=EDGE_CURVE('',#3561,#3563,#1707,.T.);
#4521=EDGE_CURVE('',#3554,#3564,#2376,.T.);
#4522=EDGE_CURVE('',#3565,#3564,#2377,.T.);
#4523=EDGE_CURVE('',#3566,#3565,#2378,.T.);
#4524=EDGE_CURVE('',#3563,#3566,#2379,.T.);
#4525=EDGE_CURVE('',#3552,#3567,#2380,.T.);
#4526=EDGE_CURVE('',#3564,#3567,#1708,.T.);
#4527=EDGE_CURVE('',#3568,#3549,#2381,.T.);
#4528=EDGE_CURVE('',#3567,#3568,#2382,.T.);
#4529=EDGE_CURVE('',#3551,#3569,#2383,.T.);
#4530=EDGE_CURVE('',#3568,#3569,#1709,.T.);
#4531=EDGE_CURVE('',#3536,#3551,#1710,.T.);
#4532=EDGE_CURVE('',#3550,#3535,#1711,.T.);
#4533=EDGE_CURVE('',#3538,#3570,#1712,.T.);
#4534=EDGE_CURVE('',#3570,#3536,#2384,.T.);
#4535=EDGE_CURVE('',#3571,#3572,#1713,.T.);
#4536=EDGE_CURVE('',#3572,#3570,#1714,.T.);
#4537=EDGE_CURVE('',#3538,#3571,#1715,.T.);
#4538=EDGE_CURVE('',#3573,#3574,#1716,.T.);
#4539=EDGE_CURVE('',#3574,#3572,#2385,.T.);
#4540=EDGE_CURVE('',#3571,#3573,#2386,.T.);
#4541=EDGE_CURVE('',#3569,#3574,#1717,.T.);
#4542=EDGE_CURVE('',#3573,#3568,#1718,.T.);
#4543=EDGE_CURVE('',#3537,#3575,#1719,.T.);
#4544=EDGE_CURVE('',#3575,#3571,#2387,.T.);
#4545=EDGE_CURVE('',#3522,#3546,#2388,.T.);
#4546=EDGE_CURVE('',#3562,#3576,#1720,.T.);
#4547=EDGE_CURVE('',#3576,#3548,#2389,.T.);
#4548=EDGE_CURVE('',#3577,#3578,#1721,.T.);
#4549=EDGE_CURVE('',#3578,#3576,#1722,.T.);
#4550=EDGE_CURVE('',#3562,#3577,#1723,.T.);
#4551=EDGE_CURVE('',#3579,#3580,#1724,.T.);
#4552=EDGE_CURVE('',#3580,#3578,#2390,.T.);
#4553=EDGE_CURVE('',#3577,#3579,#2391,.T.);
#4554=EDGE_CURVE('',#3545,#3580,#1725,.T.);
#4555=EDGE_CURVE('',#3579,#3544,#1726,.T.);
#4556=EDGE_CURVE('',#3561,#3581,#1727,.T.);
#4557=EDGE_CURVE('',#3581,#3577,#2392,.T.);
#4558=EDGE_CURVE('',#3582,#3565,#1728,.T.);
#4559=EDGE_CURVE('',#3564,#3583,#1729,.T.);
#4560=EDGE_CURVE('',#3583,#3582,#2393,.T.);
#4561=EDGE_CURVE('',#3567,#3584,#1730,.T.);
#4562=EDGE_CURVE('',#3584,#3583,#1731,.T.);
#4563=EDGE_CURVE('',#3573,#3584,#2394,.T.);
#4564=EDGE_CURVE('',#3585,#3586,#1732,.T.);
#4565=EDGE_CURVE('',#3586,#3565,#1733,.T.);
#4566=EDGE_CURVE('',#3582,#3585,#1734,.T.);
#4567=EDGE_CURVE('',#3587,#3575,#1735,.T.);
#4568=EDGE_CURVE('',#3588,#3587,#2395,.T.);
#4569=EDGE_CURVE('',#3589,#3588,#1736,.T.);
#4570=EDGE_CURVE('',#3590,#3589,#2396,.T.);
#4571=EDGE_CURVE('',#3591,#3590,#2397,.T.);
#4572=EDGE_CURVE('',#3591,#3585,#2398,.T.);
#4573=EDGE_CURVE('',#3592,#3593,#1737,.T.);
#4574=EDGE_CURVE('',#3593,#3592,#2399,.T.);
#4575=EDGE_CURVE('',#3539,#3587,#1738,.T.);
#4576=EDGE_CURVE('',#3542,#3588,#1739,.T.);
#4577=EDGE_CURVE('',#3594,#3589,#1740,.T.);
#4578=EDGE_CURVE('',#3542,#3594,#1741,.T.);
#4579=EDGE_CURVE('',#3595,#3541,#1742,.T.);
#4580=EDGE_CURVE('',#3540,#3596,#1743,.T.);
#4581=EDGE_CURVE('',#3596,#3595,#2400,.T.);
#4582=EDGE_CURVE('',#3543,#3597,#1744,.T.);
#4583=EDGE_CURVE('',#3597,#3596,#1745,.T.);
#4584=EDGE_CURVE('',#3579,#3597,#2401,.T.);
#4585=EDGE_CURVE('',#3598,#3599,#1746,.T.);
#4586=EDGE_CURVE('',#3599,#3541,#1747,.T.);
#4587=EDGE_CURVE('',#3595,#3598,#1748,.T.);
#4588=EDGE_CURVE('',#3600,#3581,#1749,.T.);
#4589=EDGE_CURVE('',#3601,#3600,#2402,.T.);
#4590=EDGE_CURVE('',#3602,#3601,#1750,.T.);
#4591=EDGE_CURVE('',#3603,#3602,#2403,.T.);
#4592=EDGE_CURVE('',#3604,#3603,#2404,.T.);
#4593=EDGE_CURVE('',#3604,#3598,#2405,.T.);
#4594=EDGE_CURVE('',#3605,#3606,#2406,.T.);
#4595=EDGE_CURVE('',#3606,#3605,#1751,.T.);
#4596=EDGE_CURVE('',#3563,#3600,#1752,.T.);
#4597=EDGE_CURVE('',#3566,#3601,#1753,.T.);
#4598=EDGE_CURVE('',#3607,#3602,#1754,.T.);
#4599=EDGE_CURVE('',#3566,#3607,#1755,.T.);
#4600=EDGE_CURVE('',#3594,#3599,#2407,.T.);
#4601=EDGE_CURVE('',#3586,#3607,#2408,.T.);
#4602=EDGE_CURVE('',#3608,#3599,#2409,.T.);
#4603=EDGE_CURVE('',#3609,#3608,#2410,.T.);
#4604=EDGE_CURVE('',#3609,#3594,#2411,.T.);
#4605=EDGE_CURVE('',#3610,#3586,#2412,.T.);
#4606=EDGE_CURVE('',#3611,#3610,#2413,.T.);
#4607=EDGE_CURVE('',#3611,#3607,#2414,.T.);
#4608=EDGE_CURVE('',#3592,#3612,#2415,.T.);
#4609=EDGE_CURVE('',#3613,#3612,#1756,.T.);
#4610=EDGE_CURVE('',#3613,#3593,#2416,.T.);
#4611=EDGE_CURVE('',#3612,#3613,#2417,.T.);
#4612=EDGE_CURVE('',#3614,#3605,#2418,.T.);
#4613=EDGE_CURVE('',#3615,#3614,#2419,.T.);
#4614=EDGE_CURVE('',#3606,#3615,#2420,.T.);
#4615=EDGE_CURVE('',#3614,#3615,#1757,.T.);
#4616=EDGE_CURVE('',#3608,#3604,#1758,.T.);
#4617=EDGE_CURVE('',#3603,#3611,#1759,.T.);
#4618=EDGE_CURVE('',#3610,#3591,#1760,.T.);
#4619=EDGE_CURVE('',#3590,#3609,#1761,.T.);
#4620=EDGE_CURVE('',#3616,#3513,#2421,.T.);
#4621=EDGE_CURVE('',#3616,#3521,#1762,.T.);
#4622=EDGE_CURVE('',#3617,#3512,#2422,.T.);
#4623=EDGE_CURVE('',#3617,#3616,#2423,.T.);
#4624=EDGE_CURVE('',#3618,#3510,#2424,.T.);
#4625=EDGE_CURVE('',#3618,#3617,#1763,.T.);
#4626=EDGE_CURVE('',#3518,#3618,#2425,.T.);
#6121=ORIENTED_EDGE('',*,*,#4428,.T.);
#6122=ORIENTED_EDGE('',*,*,#4429,.T.);
#6123=ORIENTED_EDGE('',*,*,#4430,.T.);
#6124=ORIENTED_EDGE('',*,*,#4431,.T.);
#6125=ORIENTED_EDGE('',*,*,#4432,.T.);
#6126=ORIENTED_EDGE('',*,*,#4433,.T.);
#6127=ORIENTED_EDGE('',*,*,#4434,.T.);
#6128=ORIENTED_EDGE('',*,*,#4435,.T.);
#6129=ORIENTED_EDGE('',*,*,#4432,.F.);
#6130=ORIENTED_EDGE('',*,*,#4430,.F.);
#6131=ORIENTED_EDGE('',*,*,#4436,.T.);
#6132=ORIENTED_EDGE('',*,*,#4437,.T.);
#6133=ORIENTED_EDGE('',*,*,#4438,.T.);
#6134=ORIENTED_EDGE('',*,*,#4439,.T.);
#6135=ORIENTED_EDGE('',*,*,#4440,.T.);
#6136=ORIENTED_EDGE('',*,*,#4437,.F.);
#6137=ORIENTED_EDGE('',*,*,#4434,.F.);
#6138=ORIENTED_EDGE('',*,*,#4441,.T.);
#6139=ORIENTED_EDGE('',*,*,#4442,.T.);
#6140=ORIENTED_EDGE('',*,*,#4443,.T.);
#6141=ORIENTED_EDGE('',*,*,#4444,.T.);
#6142=ORIENTED_EDGE('',*,*,#4445,.T.);
#6143=ORIENTED_EDGE('',*,*,#4442,.F.);
#6144=ORIENTED_EDGE('',*,*,#4439,.F.);
#6145=ORIENTED_EDGE('',*,*,#4446,.T.);
#6146=ORIENTED_EDGE('',*,*,#4428,.F.);
#6147=ORIENTED_EDGE('',*,*,#4444,.F.);
#6148=ORIENTED_EDGE('',*,*,#4447,.T.);
#6149=ORIENTED_EDGE('',*,*,#4436,.F.);
#6150=ORIENTED_EDGE('',*,*,#4448,.F.);
#6151=ORIENTED_EDGE('',*,*,#4449,.T.);
#6152=ORIENTED_EDGE('',*,*,#4450,.T.);
#6153=ORIENTED_EDGE('',*,*,#4429,.F.);
#6154=ORIENTED_EDGE('',*,*,#4451,.F.);
#6155=ORIENTED_EDGE('',*,*,#4452,.T.);
#6156=ORIENTED_EDGE('',*,*,#4448,.T.);
#6157=ORIENTED_EDGE('',*,*,#4447,.F.);
#6158=ORIENTED_EDGE('',*,*,#4453,.F.);
#6159=ORIENTED_EDGE('',*,*,#4454,.T.);
#6160=ORIENTED_EDGE('',*,*,#4451,.T.);
#6161=ORIENTED_EDGE('',*,*,#4443,.F.);
#6162=ORIENTED_EDGE('',*,*,#4455,.F.);
#6163=ORIENTED_EDGE('',*,*,#4456,.T.);
#6164=ORIENTED_EDGE('',*,*,#4453,.T.);
#6165=ORIENTED_EDGE('',*,*,#4431,.F.);
#6166=ORIENTED_EDGE('',*,*,#4435,.F.);
#6167=ORIENTED_EDGE('',*,*,#4440,.F.);
#6168=ORIENTED_EDGE('',*,*,#4445,.F.);
#6169=ORIENTED_EDGE('',*,*,#4457,.T.);
#6170=ORIENTED_EDGE('',*,*,#4458,.T.);
#6171=ORIENTED_EDGE('',*,*,#4459,.T.);
#6172=ORIENTED_EDGE('',*,*,#4460,.T.);
#6173=ORIENTED_EDGE('',*,*,#4461,.T.);
#6174=ORIENTED_EDGE('',*,*,#4462,.T.);
#6175=ORIENTED_EDGE('',*,*,#4458,.F.);
#6176=ORIENTED_EDGE('',*,*,#4463,.T.);
#6177=ORIENTED_EDGE('',*,*,#4464,.T.);
#6178=ORIENTED_EDGE('',*,*,#4465,.T.);
#6179=ORIENTED_EDGE('',*,*,#4461,.F.);
#6180=ORIENTED_EDGE('',*,*,#4466,.T.);
#6181=ORIENTED_EDGE('',*,*,#4467,.T.);
#6182=ORIENTED_EDGE('',*,*,#4468,.T.);
#6183=ORIENTED_EDGE('',*,*,#4464,.F.);
#6184=ORIENTED_EDGE('',*,*,#4469,.T.);
#6185=ORIENTED_EDGE('',*,*,#4470,.T.);
#6186=ORIENTED_EDGE('',*,*,#4471,.T.);
#6187=ORIENTED_EDGE('',*,*,#4467,.F.);
#6188=ORIENTED_EDGE('',*,*,#4472,.T.);
#6189=ORIENTED_EDGE('',*,*,#4473,.T.);
#6190=ORIENTED_EDGE('',*,*,#4474,.T.);
#6191=ORIENTED_EDGE('',*,*,#4470,.F.);
#6192=ORIENTED_EDGE('',*,*,#4475,.T.);
#6193=ORIENTED_EDGE('',*,*,#4473,.F.);
#6194=ORIENTED_EDGE('',*,*,#4476,.T.);
#6195=ORIENTED_EDGE('',*,*,#4477,.T.);
#6196=ORIENTED_EDGE('',*,*,#4475,.F.);
#6197=ORIENTED_EDGE('',*,*,#4478,.T.);
#6198=ORIENTED_EDGE('',*,*,#4479,.F.);
#6199=ORIENTED_EDGE('',*,*,#4480,.F.);
#6200=ORIENTED_EDGE('',*,*,#4472,.F.);
#6201=ORIENTED_EDGE('',*,*,#4481,.F.);
#6202=ORIENTED_EDGE('',*,*,#4482,.F.);
#6203=ORIENTED_EDGE('',*,*,#4478,.F.);
#6204=ORIENTED_EDGE('',*,*,#4469,.F.);
#6205=ORIENTED_EDGE('',*,*,#4483,.T.);
#6206=ORIENTED_EDGE('',*,*,#4484,.F.);
#6207=ORIENTED_EDGE('',*,*,#4485,.T.);
#6208=ORIENTED_EDGE('',*,*,#4486,.F.);
#6209=ORIENTED_EDGE('',*,*,#4481,.T.);
#6210=ORIENTED_EDGE('',*,*,#4466,.F.);
#6211=ORIENTED_EDGE('',*,*,#4487,.F.);
#6212=ORIENTED_EDGE('',*,*,#4488,.F.);
#6213=ORIENTED_EDGE('',*,*,#4483,.F.);
#6214=ORIENTED_EDGE('',*,*,#4463,.F.);
#6215=ORIENTED_EDGE('',*,*,#4489,.F.);
#6216=ORIENTED_EDGE('',*,*,#4490,.F.);
#6217=ORIENTED_EDGE('',*,*,#4487,.T.);
#6218=ORIENTED_EDGE('',*,*,#4460,.F.);
#6219=ORIENTED_EDGE('',*,*,#4491,.T.);
#6220=ORIENTED_EDGE('',*,*,#4492,.F.);
#6221=ORIENTED_EDGE('',*,*,#4489,.T.);
#6222=ORIENTED_EDGE('',*,*,#4459,.F.);
#6223=ORIENTED_EDGE('',*,*,#4493,.T.);
#6224=ORIENTED_EDGE('',*,*,#4494,.T.);
#6225=ORIENTED_EDGE('',*,*,#4495,.F.);
#6226=ORIENTED_EDGE('',*,*,#4496,.T.);
#6227=ORIENTED_EDGE('',*,*,#4497,.T.);
#6228=ORIENTED_EDGE('',*,*,#4498,.T.);
#6229=ORIENTED_EDGE('',*,*,#4499,.T.);
#6230=ORIENTED_EDGE('',*,*,#4500,.T.);
#6231=ORIENTED_EDGE('',*,*,#4501,.T.);
#6232=ORIENTED_EDGE('',*,*,#4497,.F.);
#6233=ORIENTED_EDGE('',*,*,#4502,.T.);
#6234=ORIENTED_EDGE('',*,*,#4503,.T.);
#6235=ORIENTED_EDGE('',*,*,#4504,.T.);
#6236=ORIENTED_EDGE('',*,*,#4500,.F.);
#6237=ORIENTED_EDGE('',*,*,#4505,.T.);
#6238=ORIENTED_EDGE('',*,*,#4506,.T.);
#6239=ORIENTED_EDGE('',*,*,#4507,.T.);
#6240=ORIENTED_EDGE('',*,*,#4503,.F.);
#6241=ORIENTED_EDGE('',*,*,#4508,.T.);
#6242=ORIENTED_EDGE('',*,*,#4509,.T.);
#6243=ORIENTED_EDGE('',*,*,#4510,.T.);
#6244=ORIENTED_EDGE('',*,*,#4506,.F.);
#6245=ORIENTED_EDGE('',*,*,#4511,.T.);
#6246=ORIENTED_EDGE('',*,*,#4512,.T.);
#6247=ORIENTED_EDGE('',*,*,#4513,.T.);
#6248=ORIENTED_EDGE('',*,*,#4509,.F.);
#6249=ORIENTED_EDGE('',*,*,#4514,.T.);
#6250=ORIENTED_EDGE('',*,*,#4512,.F.);
#6251=ORIENTED_EDGE('',*,*,#4515,.T.);
#6252=ORIENTED_EDGE('',*,*,#4495,.T.);
#6253=ORIENTED_EDGE('',*,*,#4514,.F.);
#6254=ORIENTED_EDGE('',*,*,#4516,.F.);
#6255=ORIENTED_EDGE('',*,*,#4517,.F.);
#6256=ORIENTED_EDGE('',*,*,#4518,.F.);
#6257=ORIENTED_EDGE('',*,*,#4511,.F.);
#6258=ORIENTED_EDGE('',*,*,#4519,.F.);
#6259=ORIENTED_EDGE('',*,*,#4520,.F.);
#6260=ORIENTED_EDGE('',*,*,#4516,.T.);
#6261=ORIENTED_EDGE('',*,*,#4508,.F.);
#6262=ORIENTED_EDGE('',*,*,#4521,.T.);
#6263=ORIENTED_EDGE('',*,*,#4522,.F.);
#6264=ORIENTED_EDGE('',*,*,#4523,.F.);
#6265=ORIENTED_EDGE('',*,*,#4524,.F.);
#6266=ORIENTED_EDGE('',*,*,#4519,.T.);
#6267=ORIENTED_EDGE('',*,*,#4505,.F.);
#6268=ORIENTED_EDGE('',*,*,#4525,.T.);
#6269=ORIENTED_EDGE('',*,*,#4526,.F.);
#6270=ORIENTED_EDGE('',*,*,#4521,.F.);
#6271=ORIENTED_EDGE('',*,*,#4502,.F.);
#6272=ORIENTED_EDGE('',*,*,#4527,.F.);
#6273=ORIENTED_EDGE('',*,*,#4528,.F.);
#6274=ORIENTED_EDGE('',*,*,#4525,.F.);
#6275=ORIENTED_EDGE('',*,*,#4499,.F.);
#6276=ORIENTED_EDGE('',*,*,#4529,.T.);
#6277=ORIENTED_EDGE('',*,*,#4530,.F.);
#6278=ORIENTED_EDGE('',*,*,#4527,.T.);
#6279=ORIENTED_EDGE('',*,*,#4477,.F.);
#6280=ORIENTED_EDGE('',*,*,#4531,.T.);
#6281=ORIENTED_EDGE('',*,*,#4498,.F.);
#6282=ORIENTED_EDGE('',*,*,#4532,.T.);
#6283=ORIENTED_EDGE('',*,*,#4476,.F.);
#6284=ORIENTED_EDGE('',*,*,#4480,.T.);
#6285=ORIENTED_EDGE('',*,*,#4533,.T.);
#6286=ORIENTED_EDGE('',*,*,#4534,.T.);
#6287=ORIENTED_EDGE('',*,*,#4535,.T.);
#6288=ORIENTED_EDGE('',*,*,#4536,.T.);
#6289=ORIENTED_EDGE('',*,*,#4533,.F.);
#6290=ORIENTED_EDGE('',*,*,#4537,.T.);
#6291=ORIENTED_EDGE('',*,*,#4538,.T.);
#6292=ORIENTED_EDGE('',*,*,#4539,.T.);
#6293=ORIENTED_EDGE('',*,*,#4535,.F.);
#6294=ORIENTED_EDGE('',*,*,#4540,.T.);
#6295=ORIENTED_EDGE('',*,*,#4530,.T.);
#6296=ORIENTED_EDGE('',*,*,#4541,.T.);
#6297=ORIENTED_EDGE('',*,*,#4538,.F.);
#6298=ORIENTED_EDGE('',*,*,#4542,.T.);
#6299=ORIENTED_EDGE('',*,*,#4537,.F.);
#6300=ORIENTED_EDGE('',*,*,#4479,.T.);
#6301=ORIENTED_EDGE('',*,*,#4543,.T.);
#6302=ORIENTED_EDGE('',*,*,#4544,.T.);
#6303=ORIENTED_EDGE('',*,*,#4457,.F.);
#6304=ORIENTED_EDGE('',*,*,#4545,.T.);
#6305=ORIENTED_EDGE('',*,*,#4493,.F.);
#6306=ORIENTED_EDGE('',*,*,#4462,.F.);
#6307=ORIENTED_EDGE('',*,*,#4465,.F.);
#6308=ORIENTED_EDGE('',*,*,#4468,.F.);
#6309=ORIENTED_EDGE('',*,*,#4471,.F.);
#6310=ORIENTED_EDGE('',*,*,#4474,.F.);
#6311=ORIENTED_EDGE('',*,*,#4532,.F.);
#6312=ORIENTED_EDGE('',*,*,#4501,.F.);
#6313=ORIENTED_EDGE('',*,*,#4504,.F.);
#6314=ORIENTED_EDGE('',*,*,#4507,.F.);
#6315=ORIENTED_EDGE('',*,*,#4510,.F.);
#6316=ORIENTED_EDGE('',*,*,#4513,.F.);
#6317=ORIENTED_EDGE('',*,*,#4494,.F.);
#6318=ORIENTED_EDGE('',*,*,#4545,.F.);
#6319=ORIENTED_EDGE('',*,*,#4531,.F.);
#6320=ORIENTED_EDGE('',*,*,#4534,.F.);
#6321=ORIENTED_EDGE('',*,*,#4536,.F.);
#6322=ORIENTED_EDGE('',*,*,#4539,.F.);
#6323=ORIENTED_EDGE('',*,*,#4541,.F.);
#6324=ORIENTED_EDGE('',*,*,#4529,.F.);
#6325=ORIENTED_EDGE('',*,*,#4515,.F.);
#6326=ORIENTED_EDGE('',*,*,#4518,.T.);
#6327=ORIENTED_EDGE('',*,*,#4546,.T.);
#6328=ORIENTED_EDGE('',*,*,#4547,.T.);
#6329=ORIENTED_EDGE('',*,*,#4548,.T.);
#6330=ORIENTED_EDGE('',*,*,#4549,.T.);
#6331=ORIENTED_EDGE('',*,*,#4546,.F.);
#6332=ORIENTED_EDGE('',*,*,#4550,.T.);
#6333=ORIENTED_EDGE('',*,*,#4551,.T.);
#6334=ORIENTED_EDGE('',*,*,#4552,.T.);
#6335=ORIENTED_EDGE('',*,*,#4548,.F.);
#6336=ORIENTED_EDGE('',*,*,#4553,.T.);
#6337=ORIENTED_EDGE('',*,*,#4492,.T.);
#6338=ORIENTED_EDGE('',*,*,#4554,.T.);
#6339=ORIENTED_EDGE('',*,*,#4551,.F.);
#6340=ORIENTED_EDGE('',*,*,#4555,.T.);
#6341=ORIENTED_EDGE('',*,*,#4550,.F.);
#6342=ORIENTED_EDGE('',*,*,#4517,.T.);
#6343=ORIENTED_EDGE('',*,*,#4556,.T.);
#6344=ORIENTED_EDGE('',*,*,#4557,.T.);
#6345=ORIENTED_EDGE('',*,*,#4496,.F.);
#6346=ORIENTED_EDGE('',*,*,#4547,.F.);
#6347=ORIENTED_EDGE('',*,*,#4549,.F.);
#6348=ORIENTED_EDGE('',*,*,#4552,.F.);
#6349=ORIENTED_EDGE('',*,*,#4554,.F.);
#6350=ORIENTED_EDGE('',*,*,#4491,.F.);
#6351=ORIENTED_EDGE('',*,*,#4558,.T.);
#6352=ORIENTED_EDGE('',*,*,#4522,.T.);
#6353=ORIENTED_EDGE('',*,*,#4559,.T.);
#6354=ORIENTED_EDGE('',*,*,#4560,.T.);
#6355=ORIENTED_EDGE('',*,*,#4561,.T.);
#6356=ORIENTED_EDGE('',*,*,#4562,.T.);
#6357=ORIENTED_EDGE('',*,*,#4559,.F.);
#6358=ORIENTED_EDGE('',*,*,#4526,.T.);
#6359=ORIENTED_EDGE('',*,*,#4542,.F.);
#6360=ORIENTED_EDGE('',*,*,#4563,.T.);
#6361=ORIENTED_EDGE('',*,*,#4561,.F.);
#6362=ORIENTED_EDGE('',*,*,#4528,.T.);
#6363=ORIENTED_EDGE('',*,*,#4564,.T.);
#6364=ORIENTED_EDGE('',*,*,#4565,.T.);
#6365=ORIENTED_EDGE('',*,*,#4558,.F.);
#6366=ORIENTED_EDGE('',*,*,#4566,.T.);
#6367=ORIENTED_EDGE('',*,*,#4540,.F.);
#6368=ORIENTED_EDGE('',*,*,#4544,.F.);
#6369=ORIENTED_EDGE('',*,*,#4567,.F.);
#6370=ORIENTED_EDGE('',*,*,#4568,.F.);
#6371=ORIENTED_EDGE('',*,*,#4569,.F.);
#6372=ORIENTED_EDGE('',*,*,#4570,.F.);
#6373=ORIENTED_EDGE('',*,*,#4571,.F.);
#6374=ORIENTED_EDGE('',*,*,#4572,.T.);
#6375=ORIENTED_EDGE('',*,*,#4566,.F.);
#6376=ORIENTED_EDGE('',*,*,#4560,.F.);
#6377=ORIENTED_EDGE('',*,*,#4562,.F.);
#6378=ORIENTED_EDGE('',*,*,#4563,.F.);
#6379=ORIENTED_EDGE('',*,*,#4573,.T.);
#6380=ORIENTED_EDGE('',*,*,#4574,.T.);
#6381=ORIENTED_EDGE('',*,*,#4575,.T.);
#6382=ORIENTED_EDGE('',*,*,#4567,.T.);
#6383=ORIENTED_EDGE('',*,*,#4543,.F.);
#6384=ORIENTED_EDGE('',*,*,#4482,.T.);
#6385=ORIENTED_EDGE('',*,*,#4576,.T.);
#6386=ORIENTED_EDGE('',*,*,#4568,.T.);
#6387=ORIENTED_EDGE('',*,*,#4575,.F.);
#6388=ORIENTED_EDGE('',*,*,#4486,.T.);
#6389=ORIENTED_EDGE('',*,*,#4577,.T.);
#6390=ORIENTED_EDGE('',*,*,#4569,.T.);
#6391=ORIENTED_EDGE('',*,*,#4576,.F.);
#6392=ORIENTED_EDGE('',*,*,#4578,.T.);
#6393=ORIENTED_EDGE('',*,*,#4579,.T.);
#6394=ORIENTED_EDGE('',*,*,#4484,.T.);
#6395=ORIENTED_EDGE('',*,*,#4580,.T.);
#6396=ORIENTED_EDGE('',*,*,#4581,.T.);
#6397=ORIENTED_EDGE('',*,*,#4582,.T.);
#6398=ORIENTED_EDGE('',*,*,#4583,.T.);
#6399=ORIENTED_EDGE('',*,*,#4580,.F.);
#6400=ORIENTED_EDGE('',*,*,#4488,.T.);
#6401=ORIENTED_EDGE('',*,*,#4555,.F.);
#6402=ORIENTED_EDGE('',*,*,#4584,.T.);
#6403=ORIENTED_EDGE('',*,*,#4582,.F.);
#6404=ORIENTED_EDGE('',*,*,#4490,.T.);
#6405=ORIENTED_EDGE('',*,*,#4585,.T.);
#6406=ORIENTED_EDGE('',*,*,#4586,.T.);
#6407=ORIENTED_EDGE('',*,*,#4579,.F.);
#6408=ORIENTED_EDGE('',*,*,#4587,.T.);
#6409=ORIENTED_EDGE('',*,*,#4553,.F.);
#6410=ORIENTED_EDGE('',*,*,#4557,.F.);
#6411=ORIENTED_EDGE('',*,*,#4588,.F.);
#6412=ORIENTED_EDGE('',*,*,#4589,.F.);
#6413=ORIENTED_EDGE('',*,*,#4590,.F.);
#6414=ORIENTED_EDGE('',*,*,#4591,.F.);
#6415=ORIENTED_EDGE('',*,*,#4592,.F.);
#6416=ORIENTED_EDGE('',*,*,#4593,.T.);
#6417=ORIENTED_EDGE('',*,*,#4587,.F.);
#6418=ORIENTED_EDGE('',*,*,#4581,.F.);
#6419=ORIENTED_EDGE('',*,*,#4583,.F.);
#6420=ORIENTED_EDGE('',*,*,#4584,.F.);
#6421=ORIENTED_EDGE('',*,*,#4594,.T.);
#6422=ORIENTED_EDGE('',*,*,#4595,.T.);
#6423=ORIENTED_EDGE('',*,*,#4596,.T.);
#6424=ORIENTED_EDGE('',*,*,#4588,.T.);
#6425=ORIENTED_EDGE('',*,*,#4556,.F.);
#6426=ORIENTED_EDGE('',*,*,#4520,.T.);
#6427=ORIENTED_EDGE('',*,*,#4597,.T.);
#6428=ORIENTED_EDGE('',*,*,#4589,.T.);
#6429=ORIENTED_EDGE('',*,*,#4596,.F.);
#6430=ORIENTED_EDGE('',*,*,#4524,.T.);
#6431=ORIENTED_EDGE('',*,*,#4598,.T.);
#6432=ORIENTED_EDGE('',*,*,#4590,.T.);
#6433=ORIENTED_EDGE('',*,*,#4597,.F.);
#6434=ORIENTED_EDGE('',*,*,#4599,.T.);
#6435=ORIENTED_EDGE('',*,*,#4578,.F.);
#6436=ORIENTED_EDGE('',*,*,#4485,.F.);
#6437=ORIENTED_EDGE('',*,*,#4586,.F.);
#6438=ORIENTED_EDGE('',*,*,#4600,.F.);
#6439=ORIENTED_EDGE('',*,*,#4565,.F.);
#6440=ORIENTED_EDGE('',*,*,#4601,.T.);
#6441=ORIENTED_EDGE('',*,*,#4599,.F.);
#6442=ORIENTED_EDGE('',*,*,#4523,.T.);
#6443=ORIENTED_EDGE('',*,*,#4600,.T.);
#6444=ORIENTED_EDGE('',*,*,#4602,.F.);
#6445=ORIENTED_EDGE('',*,*,#4603,.F.);
#6446=ORIENTED_EDGE('',*,*,#4604,.T.);
#6447=ORIENTED_EDGE('',*,*,#4601,.F.);
#6448=ORIENTED_EDGE('',*,*,#4605,.F.);
#6449=ORIENTED_EDGE('',*,*,#4606,.F.);
#6450=ORIENTED_EDGE('',*,*,#4607,.T.);
#6451=ORIENTED_EDGE('',*,*,#4573,.F.);
#6452=ORIENTED_EDGE('',*,*,#4608,.T.);
#6453=ORIENTED_EDGE('',*,*,#4609,.F.);
#6454=ORIENTED_EDGE('',*,*,#4610,.T.);
#6455=ORIENTED_EDGE('',*,*,#4574,.F.);
#6456=ORIENTED_EDGE('',*,*,#4610,.F.);
#6457=ORIENTED_EDGE('',*,*,#4611,.F.);
#6458=ORIENTED_EDGE('',*,*,#4608,.F.);
#6459=ORIENTED_EDGE('',*,*,#4609,.T.);
#6460=ORIENTED_EDGE('',*,*,#4611,.T.);
#6461=ORIENTED_EDGE('',*,*,#4594,.F.);
#6462=ORIENTED_EDGE('',*,*,#4612,.F.);
#6463=ORIENTED_EDGE('',*,*,#4613,.F.);
#6464=ORIENTED_EDGE('',*,*,#4614,.F.);
#6465=ORIENTED_EDGE('',*,*,#4615,.T.);
#6466=ORIENTED_EDGE('',*,*,#4613,.T.);
#6467=ORIENTED_EDGE('',*,*,#4595,.F.);
#6468=ORIENTED_EDGE('',*,*,#4614,.T.);
#6469=ORIENTED_EDGE('',*,*,#4615,.F.);
#6470=ORIENTED_EDGE('',*,*,#4612,.T.);
#6471=ORIENTED_EDGE('',*,*,#4585,.F.);
#6472=ORIENTED_EDGE('',*,*,#4593,.F.);
#6473=ORIENTED_EDGE('',*,*,#4616,.F.);
#6474=ORIENTED_EDGE('',*,*,#4602,.T.);
#6475=ORIENTED_EDGE('',*,*,#4598,.F.);
#6476=ORIENTED_EDGE('',*,*,#4607,.F.);
#6477=ORIENTED_EDGE('',*,*,#4617,.F.);
#6478=ORIENTED_EDGE('',*,*,#4591,.T.);
#6479=ORIENTED_EDGE('',*,*,#4564,.F.);
#6480=ORIENTED_EDGE('',*,*,#4572,.F.);
#6481=ORIENTED_EDGE('',*,*,#4618,.F.);
#6482=ORIENTED_EDGE('',*,*,#4605,.T.);
#6483=ORIENTED_EDGE('',*,*,#4577,.F.);
#6484=ORIENTED_EDGE('',*,*,#4604,.F.);
#6485=ORIENTED_EDGE('',*,*,#4619,.F.);
#6486=ORIENTED_EDGE('',*,*,#4570,.T.);
#6487=ORIENTED_EDGE('',*,*,#4446,.F.);
#6488=ORIENTED_EDGE('',*,*,#4620,.F.);
#6489=ORIENTED_EDGE('',*,*,#4621,.T.);
#6490=ORIENTED_EDGE('',*,*,#4455,.T.);
#6491=ORIENTED_EDGE('',*,*,#4438,.F.);
#6492=ORIENTED_EDGE('',*,*,#4622,.F.);
#6493=ORIENTED_EDGE('',*,*,#4623,.T.);
#6494=ORIENTED_EDGE('',*,*,#4620,.T.);
#6495=ORIENTED_EDGE('',*,*,#4441,.F.);
#6496=ORIENTED_EDGE('',*,*,#4624,.F.);
#6497=ORIENTED_EDGE('',*,*,#4625,.T.);
#6498=ORIENTED_EDGE('',*,*,#4622,.T.);
#6499=ORIENTED_EDGE('',*,*,#4433,.F.);
#6500=ORIENTED_EDGE('',*,*,#4450,.F.);
#6501=ORIENTED_EDGE('',*,*,#4626,.T.);
#6502=ORIENTED_EDGE('',*,*,#4624,.T.);
#6503=ORIENTED_EDGE('',*,*,#4626,.F.);
#6504=ORIENTED_EDGE('',*,*,#4449,.F.);
#6505=ORIENTED_EDGE('',*,*,#4452,.F.);
#6506=ORIENTED_EDGE('',*,*,#4454,.F.);
#6507=ORIENTED_EDGE('',*,*,#4456,.F.);
#6508=ORIENTED_EDGE('',*,*,#4621,.F.);
#6509=ORIENTED_EDGE('',*,*,#4623,.F.);
#6510=ORIENTED_EDGE('',*,*,#4625,.F.);
#6511=ORIENTED_EDGE('',*,*,#4603,.T.);
#6512=ORIENTED_EDGE('',*,*,#4616,.T.);
#6513=ORIENTED_EDGE('',*,*,#4592,.T.);
#6514=ORIENTED_EDGE('',*,*,#4617,.T.);
#6515=ORIENTED_EDGE('',*,*,#4606,.T.);
#6516=ORIENTED_EDGE('',*,*,#4618,.T.);
#6517=ORIENTED_EDGE('',*,*,#4571,.T.);
#6518=ORIENTED_EDGE('',*,*,#4619,.T.);
#7530=CYLINDRICAL_SURFACE('',#8649,2.);
#7531=CYLINDRICAL_SURFACE('',#8652,2.);
#7532=CYLINDRICAL_SURFACE('',#8657,2.);
#7533=CYLINDRICAL_SURFACE('',#8662,2.);
#7534=CYLINDRICAL_SURFACE('',#8669,2.);
#7535=CYLINDRICAL_SURFACE('',#8672,2.00000000000001);
#7536=CYLINDRICAL_SURFACE('',#8681,0.2);
#7537=CYLINDRICAL_SURFACE('',#8688,0.2);
#7538=CYLINDRICAL_SURFACE('',#8694,0.999999999999871);
#7539=CYLINDRICAL_SURFACE('',#8697,0.999999999999871);
#7540=CYLINDRICAL_SURFACE('',#8700,0.2);
#7541=CYLINDRICAL_SURFACE('',#8711,0.2);
#7542=CYLINDRICAL_SURFACE('',#8718,0.2);
#7543=CYLINDRICAL_SURFACE('',#8723,0.999999999999871);
#7544=CYLINDRICAL_SURFACE('',#8726,0.999999999999871);
#7545=CYLINDRICAL_SURFACE('',#8729,0.2);
#7546=CYLINDRICAL_SURFACE('',#8734,0.2);
#7547=CYLINDRICAL_SURFACE('',#8739,0.2);
#7548=CYLINDRICAL_SURFACE('',#8743,0.4);
#7549=CYLINDRICAL_SURFACE('',#8745,9.);
#7550=CYLINDRICAL_SURFACE('',#8747,0.2);
#7551=CYLINDRICAL_SURFACE('',#8752,0.2);
#7552=CYLINDRICAL_SURFACE('',#8756,0.4);
#7553=CYLINDRICAL_SURFACE('',#8759,0.4);
#7554=CYLINDRICAL_SURFACE('',#8765,0.4);
#7555=CYLINDRICAL_SURFACE('',#8775,0.4);
#7556=CYLINDRICAL_SURFACE('',#8779,0.4);
#7557=CYLINDRICAL_SURFACE('',#8785,0.4);
#7558=CYLINDRICAL_SURFACE('',#8795,0.4);
#7559=CYLINDRICAL_SURFACE('',#8799,0.800000000000058);
#7560=CYLINDRICAL_SURFACE('',#8800,0.800000000000058);
#7561=CYLINDRICAL_SURFACE('',#8803,2.98575787723652);
#7562=CYLINDRICAL_SURFACE('',#8810,2.98575787723652);
#7563=CYLINDRICAL_SURFACE('',#8811,0.399999999999998);
#7564=CYLINDRICAL_SURFACE('',#8813,0.4);
#7565=CYLINDRICAL_SURFACE('',#8815,0.400000000000004);
#7566=CYLINDRICAL_SURFACE('',#8817,0.4);
#7567=CYLINDRICAL_SURFACE('',#8819,2.);
#7568=CYLINDRICAL_SURFACE('',#8822,2.);
#7833=ADVANCED_FACE('',(#671),#7530,.T.);
#7834=ADVANCED_FACE('',(#672),#7531,.T.);
#7835=ADVANCED_FACE('',(#673),#202,.T.);
#7836=ADVANCED_FACE('',(#674),#7532,.T.);
#7837=ADVANCED_FACE('',(#675),#203,.T.);
#7838=ADVANCED_FACE('',(#676),#7533,.T.);
#7839=ADVANCED_FACE('',(#677),#204,.T.);
#7840=ADVANCED_FACE('',(#678),#205,.T.);
#7841=ADVANCED_FACE('',(#679),#7534,.T.);
#7842=ADVANCED_FACE('',(#680),#370,.T.);
#7843=ADVANCED_FACE('',(#681),#7535,.T.);
#7844=ADVANCED_FACE('',(#682),#371,.T.);
#7845=ADVANCED_FACE('',(#683,#158),#372,.T.);
#7846=ADVANCED_FACE('',(#684),#206,.T.);
#7847=ADVANCED_FACE('',(#685),#7536,.T.);
#7848=ADVANCED_FACE('',(#686),#70,.F.);
#7849=ADVANCED_FACE('',(#687),#71,.F.);
#7850=ADVANCED_FACE('',(#688),#72,.F.);
#7851=ADVANCED_FACE('',(#689),#7537,.T.);
#7852=ADVANCED_FACE('',(#690),#207,.T.);
#7853=ADVANCED_FACE('',(#691),#373,.F.);
#7854=ADVANCED_FACE('',(#692),#7538,.F.);
#7855=ADVANCED_FACE('',(#693),#374,.F.);
#7856=ADVANCED_FACE('',(#694),#7539,.F.);
#7857=ADVANCED_FACE('',(#695),#375,.F.);
#7858=ADVANCED_FACE('',(#696),#7540,.T.);
#7859=ADVANCED_FACE('',(#697),#220,.T.);
#7860=ADVANCED_FACE('',(#698),#208,.T.);
#7861=ADVANCED_FACE('',(#699),#7541,.T.);
#7862=ADVANCED_FACE('',(#700),#73,.F.);
#7863=ADVANCED_FACE('',(#701),#74,.F.);
#7864=ADVANCED_FACE('',(#702),#75,.F.);
#7865=ADVANCED_FACE('',(#703),#7542,.T.);
#7866=ADVANCED_FACE('',(#704),#209,.T.);
#7867=ADVANCED_FACE('',(#705),#376,.F.);
#7868=ADVANCED_FACE('',(#706),#7543,.F.);
#7869=ADVANCED_FACE('',(#707),#377,.F.);
#7870=ADVANCED_FACE('',(#708),#7544,.F.);
#7871=ADVANCED_FACE('',(#709),#378,.F.);
#7872=ADVANCED_FACE('',(#710),#7545,.T.);
#7873=ADVANCED_FACE('',(#711),#221,.T.);
#7874=ADVANCED_FACE('',(#712),#7546,.T.);
#7875=ADVANCED_FACE('',(#713),#188,.F.);
#7876=ADVANCED_FACE('',(#714),#7547,.T.);
#7877=ADVANCED_FACE('',(#715),#189,.F.);
#7878=ADVANCED_FACE('',(#716),#7548,.T.);
#7879=ADVANCED_FACE('',(#717),#7549,.F.);
#7880=ADVANCED_FACE('',(#718),#379,.F.);
#7881=ADVANCED_FACE('',(#719),#7550,.T.);
#7882=ADVANCED_FACE('',(#720),#190,.F.);
#7883=ADVANCED_FACE('',(#721),#7551,.T.);
#7884=ADVANCED_FACE('',(#722),#191,.F.);
#7885=ADVANCED_FACE('',(#723),#7552,.T.);
#7886=ADVANCED_FACE('',(#724),#380,.F.);
#7887=ADVANCED_FACE('',(#725),#7553,.T.);
#7888=ADVANCED_FACE('',(#726),#222,.T.);
#7889=ADVANCED_FACE('',(#727),#7554,.T.);
#7890=ADVANCED_FACE('',(#728),#192,.F.);
#7891=ADVANCED_FACE('',(#729,#159),#381,.T.);
#7892=ADVANCED_FACE('',(#730),#223,.T.);
#7893=ADVANCED_FACE('',(#731),#7555,.T.);
#7894=ADVANCED_FACE('',(#732),#193,.F.);
#7895=ADVANCED_FACE('',(#733),#7556,.T.);
#7896=ADVANCED_FACE('',(#734),#224,.T.);
#7897=ADVANCED_FACE('',(#735),#7557,.T.);
#7898=ADVANCED_FACE('',(#736),#194,.F.);
#7899=ADVANCED_FACE('',(#737,#160),#382,.T.);
#7900=ADVANCED_FACE('',(#738),#225,.T.);
#7901=ADVANCED_FACE('',(#739),#7558,.T.);
#7902=ADVANCED_FACE('',(#740),#195,.F.);
#7903=ADVANCED_FACE('',(#741),#7559,.T.);
#7904=ADVANCED_FACE('',(#742),#7560,.T.);
#7905=ADVANCED_FACE('',(#743),#383,.T.);
#7906=ADVANCED_FACE('',(#744),#384,.T.);
#7907=ADVANCED_FACE('',(#745),#7561,.T.);
#7908=ADVANCED_FACE('',(#746),#385,.T.);
#7909=ADVANCED_FACE('',(#747),#386,.T.);
#7910=ADVANCED_FACE('',(#748),#387,.T.);
#7911=ADVANCED_FACE('',(#749),#388,.F.);
#7912=ADVANCED_FACE('',(#750),#7562,.T.);
#7913=ADVANCED_FACE('',(#751),#7563,.T.);
#7914=ADVANCED_FACE('',(#752),#7564,.T.);
#7915=ADVANCED_FACE('',(#753),#7565,.T.);
#7916=ADVANCED_FACE('',(#754),#7566,.T.);
#7917=ADVANCED_FACE('',(#755),#7567,.T.);
#7918=ADVANCED_FACE('',(#756),#389,.T.);
#7919=ADVANCED_FACE('',(#757),#7568,.T.);
#7920=ADVANCED_FACE('',(#758),#390,.T.);
#7921=ADVANCED_FACE('',(#759,#161),#391,.F.);
#8118=CLOSED_SHELL('',(#7833,#7834,#7835,#7836,#7837,#7838,#7839,#7840,
#7841,#7842,#7843,#7844,#7845,#7846,#7847,#7848,#7849,#7850,#7851,#7852,
#7853,#7854,#7855,#7856,#7857,#7858,#7859,#7860,#7861,#7862,#7863,#7864,
#7865,#7866,#7867,#7868,#7869,#7870,#7871,#7872,#7873,#7874,#7875,#7876,
#7877,#7878,#7879,#7880,#7881,#7882,#7883,#7884,#7885,#7886,#7887,#7888,
#7889,#7890,#7891,#7892,#7893,#7894,#7895,#7896,#7897,#7898,#7899,#7900,
#7901,#7902,#7903,#7904,#7905,#7906,#7907,#7908,#7909,#7910,#7911,#7912,
#7913,#7914,#7915,#7916,#7917,#7918,#7919,#7920,#7921));
#8648=AXIS2_PLACEMENT_3D('',#12957,#10342,#10343);
#8649=AXIS2_PLACEMENT_3D('',#12958,#10344,#10345);
#8650=AXIS2_PLACEMENT_3D('',#12961,#10346,#10347);
#8651=AXIS2_PLACEMENT_3D('',#12965,#10349,#10350);
#8652=AXIS2_PLACEMENT_3D('',#12967,#10352,#10353);
#8653=AXIS2_PLACEMENT_3D('',#12969,#10354,#10355);
#8654=AXIS2_PLACEMENT_3D('',#12973,#10357,#10358);
#8655=AXIS2_PLACEMENT_3D('',#12975,#10360,#10361);
#8656=AXIS2_PLACEMENT_3D('',#12976,#10362,#10363);
#8657=AXIS2_PLACEMENT_3D('',#12977,#10364,#10365);
#8658=AXIS2_PLACEMENT_3D('',#12979,#10366,#10367);
#8659=AXIS2_PLACEMENT_3D('',#12983,#10369,#10370);
#8660=AXIS2_PLACEMENT_3D('',#12985,#10372,#10373);
#8661=AXIS2_PLACEMENT_3D('',#12986,#10374,#10375);
#8662=AXIS2_PLACEMENT_3D('',#12987,#10376,#10377);
#8663=AXIS2_PLACEMENT_3D('',#12989,#10378,#10379);
#8664=AXIS2_PLACEMENT_3D('',#12992,#10381,#10382);
#8665=AXIS2_PLACEMENT_3D('',#12994,#10384,#10385);
#8666=AXIS2_PLACEMENT_3D('',#12995,#10386,#10387);
#8667=AXIS2_PLACEMENT_3D('',#12996,#10388,#10389);
#8668=AXIS2_PLACEMENT_3D('',#12997,#10390,#10391);
#8669=AXIS2_PLACEMENT_3D('',#12998,#10392,#10393);
#8670=AXIS2_PLACEMENT_3D('',#13002,#10395,#10396);
#8671=AXIS2_PLACEMENT_3D('',#13004,#10398,#10399);
#8672=AXIS2_PLACEMENT_3D('',#13008,#10402,#10403);
#8673=AXIS2_PLACEMENT_3D('',#13011,#10405,#10406);
#8674=AXIS2_PLACEMENT_3D('',#13012,#10407,#10408);
#8675=AXIS2_PLACEMENT_3D('',#13016,#10411,#10412);
#8676=AXIS2_PLACEMENT_3D('',#13018,#10413,#10414);
#8677=AXIS2_PLACEMENT_3D('',#13019,#10415,#10416);
#8678=AXIS2_PLACEMENT_3D('',#13022,#10417,#10418);
#8679=AXIS2_PLACEMENT_3D('',#13024,#10419,#10420);
#8680=AXIS2_PLACEMENT_3D('',#13025,#10421,#10422);
#8681=AXIS2_PLACEMENT_3D('',#13026,#10423,#10424);
#8682=AXIS2_PLACEMENT_3D('',#13029,#10425,#10426);
#8683=AXIS2_PLACEMENT_3D('',#13069,#10429,#10430);
#8684=AXIS2_PLACEMENT_3D('',#13124,#10431,#10432);
#8685=AXIS2_PLACEMENT_3D('',#13125,#10433,#10434);
#8686=AXIS2_PLACEMENT_3D('',#13126,#10435,#10436);
#8687=AXIS2_PLACEMENT_3D('',#13164,#10437,#10438);
#8688=AXIS2_PLACEMENT_3D('',#13175,#10439,#10440);
#8689=AXIS2_PLACEMENT_3D('',#13178,#10441,#10442);
#8690=AXIS2_PLACEMENT_3D('',#13181,#10445,#10446);
#8691=AXIS2_PLACEMENT_3D('',#13183,#10447,#10448);
#8692=AXIS2_PLACEMENT_3D('',#13184,#10449,#10450);
#8693=AXIS2_PLACEMENT_3D('',#13185,#10451,#10452);
#8694=AXIS2_PLACEMENT_3D('',#13191,#10456,#10457);
#8695=AXIS2_PLACEMENT_3D('',#13194,#10459,#10460);
#8696=AXIS2_PLACEMENT_3D('',#13195,#10461,#10462);
#8697=AXIS2_PLACEMENT_3D('',#13203,#10467,#10468);
#8698=AXIS2_PLACEMENT_3D('',#13206,#10470,#10471);
#8699=AXIS2_PLACEMENT_3D('',#13207,#10472,#10473);
#8700=AXIS2_PLACEMENT_3D('',#13211,#10476,#10477);
#8701=AXIS2_PLACEMENT_3D('',#13214,#10479,#10480);
#8702=AXIS2_PLACEMENT_3D('',#13215,#10481,#10482);
#8703=AXIS2_PLACEMENT_3D('',#13217,#10483,#10484);
#8704=AXIS2_PLACEMENT_3D('',#13219,#10485,#10486);
#8705=AXIS2_PLACEMENT_3D('',#13221,#10487,#10488);
#8706=AXIS2_PLACEMENT_3D('',#13222,#10489,#10490);
#8707=AXIS2_PLACEMENT_3D('',#13223,#10491,#10492);
#8708=AXIS2_PLACEMENT_3D('',#13226,#10493,#10494);
#8709=AXIS2_PLACEMENT_3D('',#13228,#10495,#10496);
#8710=AXIS2_PLACEMENT_3D('',#13229,#10497,#10498);
#8711=AXIS2_PLACEMENT_3D('',#13230,#10499,#10500);
#8712=AXIS2_PLACEMENT_3D('',#13233,#10501,#10502);
#8713=AXIS2_PLACEMENT_3D('',#13273,#10505,#10506);
#8714=AXIS2_PLACEMENT_3D('',#13328,#10507,#10508);
#8715=AXIS2_PLACEMENT_3D('',#13329,#10509,#10510);
#8716=AXIS2_PLACEMENT_3D('',#13330,#10511,#10512);
#8717=AXIS2_PLACEMENT_3D('',#13368,#10513,#10514);
#8718=AXIS2_PLACEMENT_3D('',#13379,#10515,#10516);
#8719=AXIS2_PLACEMENT_3D('',#13381,#10517,#10518);
#8720=AXIS2_PLACEMENT_3D('',#13384,#10521,#10522);
#8721=AXIS2_PLACEMENT_3D('',#13385,#10523,#10524);
#8722=AXIS2_PLACEMENT_3D('',#13386,#10525,#10526);
#8723=AXIS2_PLACEMENT_3D('',#13392,#10530,#10531);
#8724=AXIS2_PLACEMENT_3D('',#13395,#10533,#10534);
#8725=AXIS2_PLACEMENT_3D('',#13396,#10535,#10536);
#8726=AXIS2_PLACEMENT_3D('',#13404,#10541,#10542);
#8727=AXIS2_PLACEMENT_3D('',#13407,#10544,#10545);
#8728=AXIS2_PLACEMENT_3D('',#13408,#10546,#10547);
#8729=AXIS2_PLACEMENT_3D('',#13412,#10550,#10551);
#8730=AXIS2_PLACEMENT_3D('',#13415,#10553,#10554);
#8731=AXIS2_PLACEMENT_3D('',#13416,#10555,#10556);
#8732=AXIS2_PLACEMENT_3D('',#13417,#10557,#10558);
#8733=AXIS2_PLACEMENT_3D('',#13418,#10559,#10560);
#8734=AXIS2_PLACEMENT_3D('',#13419,#10561,#10562);
#8735=AXIS2_PLACEMENT_3D('',#13421,#10563,#10564);
#8736=AXIS2_PLACEMENT_3D('',#13434,#10566,#10567);
#8737=AXIS2_PLACEMENT_3D('',#13435,#10568,#10569);
#8738=AXIS2_PLACEMENT_3D('',#13436,#10570,#10571);
#8739=AXIS2_PLACEMENT_3D('',#13437,#10572,#10573);
#8740=AXIS2_PLACEMENT_3D('',#13440,#10574,#10575);
#8741=AXIS2_PLACEMENT_3D('',#13452,#10578,#10579);
#8742=AXIS2_PLACEMENT_3D('',#13453,#10580,#10581);
#8743=AXIS2_PLACEMENT_3D('',#13454,#10582,#10583);
#8744=AXIS2_PLACEMENT_3D('',#13456,#10584,#10585);
#8745=AXIS2_PLACEMENT_3D('',#13458,#10587,#10588);
#8746=AXIS2_PLACEMENT_3D('',#13460,#10590,#10591);
#8747=AXIS2_PLACEMENT_3D('',#13461,#10592,#10593);
#8748=AXIS2_PLACEMENT_3D('',#13463,#10594,#10595);
#8749=AXIS2_PLACEMENT_3D('',#13476,#10597,#10598);
#8750=AXIS2_PLACEMENT_3D('',#13477,#10599,#10600);
#8751=AXIS2_PLACEMENT_3D('',#13478,#10601,#10602);
#8752=AXIS2_PLACEMENT_3D('',#13479,#10603,#10604);
#8753=AXIS2_PLACEMENT_3D('',#13482,#10605,#10606);
#8754=AXIS2_PLACEMENT_3D('',#13494,#10609,#10610);
#8755=AXIS2_PLACEMENT_3D('',#13495,#10611,#10612);
#8756=AXIS2_PLACEMENT_3D('',#13496,#10613,#10614);
#8757=AXIS2_PLACEMENT_3D('',#13498,#10615,#10616);
#8758=AXIS2_PLACEMENT_3D('',#13500,#10618,#10619);
#8759=AXIS2_PLACEMENT_3D('',#13501,#10620,#10621);
#8760=AXIS2_PLACEMENT_3D('',#13503,#10622,#10623);
#8761=AXIS2_PLACEMENT_3D('',#13505,#10624,#10625);
#8762=AXIS2_PLACEMENT_3D('',#13507,#10627,#10628);
#8763=AXIS2_PLACEMENT_3D('',#13509,#10629,#10630);
#8764=AXIS2_PLACEMENT_3D('',#13510,#10631,#10632);
#8765=AXIS2_PLACEMENT_3D('',#13511,#10633,#10634);
#8766=AXIS2_PLACEMENT_3D('',#13524,#10636,#10637);
#8767=AXIS2_PLACEMENT_3D('',#13525,#10638,#10639);
#8768=AXIS2_PLACEMENT_3D('',#13526,#10640,#10641);
#8769=AXIS2_PLACEMENT_3D('',#13527,#10642,#10643);
#8770=AXIS2_PLACEMENT_3D('',#13529,#10644,#10645);
#8771=AXIS2_PLACEMENT_3D('',#13533,#10647,#10648);
#8772=AXIS2_PLACEMENT_3D('',#13541,#10652,#10653);
#8773=AXIS2_PLACEMENT_3D('',#13543,#10655,#10656);
#8774=AXIS2_PLACEMENT_3D('',#13544,#10657,#10658);
#8775=AXIS2_PLACEMENT_3D('',#13545,#10659,#10660);
#8776=AXIS2_PLACEMENT_3D('',#13546,#10661,#10662);
#8777=AXIS2_PLACEMENT_3D('',#13557,#10663,#10664);
#8778=AXIS2_PLACEMENT_3D('',#13558,#10665,#10666);
#8779=AXIS2_PLACEMENT_3D('',#13559,#10667,#10668);
#8780=AXIS2_PLACEMENT_3D('',#13561,#10669,#10670);
#8781=AXIS2_PLACEMENT_3D('',#13563,#10671,#10672);
#8782=AXIS2_PLACEMENT_3D('',#13565,#10674,#10675);
#8783=AXIS2_PLACEMENT_3D('',#13567,#10676,#10677);
#8784=AXIS2_PLACEMENT_3D('',#13568,#10678,#10679);
#8785=AXIS2_PLACEMENT_3D('',#13569,#10680,#10681);
#8786=AXIS2_PLACEMENT_3D('',#13582,#10683,#10684);
#8787=AXIS2_PLACEMENT_3D('',#13583,#10685,#10686);
#8788=AXIS2_PLACEMENT_3D('',#13584,#10687,#10688);
#8789=AXIS2_PLACEMENT_3D('',#13585,#10689,#10690);
#8790=AXIS2_PLACEMENT_3D('',#13587,#10691,#10692);
#8791=AXIS2_PLACEMENT_3D('',#13591,#10694,#10695);
#8792=AXIS2_PLACEMENT_3D('',#13600,#10700,#10701);
#8793=AXIS2_PLACEMENT_3D('',#13601,#10702,#10703);
#8794=AXIS2_PLACEMENT_3D('',#13602,#10704,#10705);
#8795=AXIS2_PLACEMENT_3D('',#13603,#10706,#10707);
#8796=AXIS2_PLACEMENT_3D('',#13604,#10708,#10709);
#8797=AXIS2_PLACEMENT_3D('',#13615,#10710,#10711);
#8798=AXIS2_PLACEMENT_3D('',#13616,#10712,#10713);
#8799=AXIS2_PLACEMENT_3D('',#13617,#10714,#10715);
#8800=AXIS2_PLACEMENT_3D('',#13619,#10717,#10718);
#8801=AXIS2_PLACEMENT_3D('',#13621,#10720,#10721);
#8802=AXIS2_PLACEMENT_3D('',#13627,#10725,#10726);
#8803=AXIS2_PLACEMENT_3D('',#13633,#10730,#10731);
#8804=AXIS2_PLACEMENT_3D('',#13637,#10733,#10734);
#8805=AXIS2_PLACEMENT_3D('',#13639,#10736,#10737);
#8806=AXIS2_PLACEMENT_3D('',#13641,#10739,#10740);
#8807=AXIS2_PLACEMENT_3D('',#13642,#10741,#10742);
#8808=AXIS2_PLACEMENT_3D('',#13648,#10746,#10747);
#8809=AXIS2_PLACEMENT_3D('',#13649,#10748,#10749);
#8810=AXIS2_PLACEMENT_3D('',#13650,#10750,#10751);
#8811=AXIS2_PLACEMENT_3D('',#13651,#10752,#10753);
#8812=AXIS2_PLACEMENT_3D('',#13652,#10754,#10755);
#8813=AXIS2_PLACEMENT_3D('',#13653,#10756,#10757);
#8814=AXIS2_PLACEMENT_3D('',#13654,#10758,#10759);
#8815=AXIS2_PLACEMENT_3D('',#13655,#10760,#10761);
#8816=AXIS2_PLACEMENT_3D('',#13656,#10762,#10763);
#8817=AXIS2_PLACEMENT_3D('',#13657,#10764,#10765);
#8818=AXIS2_PLACEMENT_3D('',#13658,#10766,#10767);
#8819=AXIS2_PLACEMENT_3D('',#13659,#10768,#10769);
#8820=AXIS2_PLACEMENT_3D('',#13662,#10771,#10772);
#8821=AXIS2_PLACEMENT_3D('',#13663,#10773,#10774);
#8822=AXIS2_PLACEMENT_3D('',#13667,#10777,#10778);
#8823=AXIS2_PLACEMENT_3D('',#13670,#10780,#10781);
#8824=AXIS2_PLACEMENT_3D('',#13671,#10782,#10783);
#8825=AXIS2_PLACEMENT_3D('',#13673,#10785,#10786);
#10342=DIRECTION('axis',(0.,0.,1.));
#10343=DIRECTION('refdir',(1.,0.,0.));
#10344=DIRECTION('center_axis',(0.,1.,0.));
#10345=DIRECTION('ref_axis',(0.707106781186555,0.,0.70710678118654));
#10346=DIRECTION('center_axis',(0.,1.,0.));
#10347=DIRECTION('ref_axis',(0.,0.,1.));
#10348=DIRECTION('',(0.,1.,0.));
#10349=DIRECTION('center_axis',(0.,-1.,0.));
#10350=DIRECTION('ref_axis',(1.,0.,0.));
#10351=DIRECTION('',(0.,-1.,0.));
#10352=DIRECTION('center_axis',(-1.,0.,0.));
#10353=DIRECTION('ref_axis',(0.,0.707106781186555,0.70710678118654));
#10354=DIRECTION('center_axis',(-1.,0.,0.));
#10355=DIRECTION('ref_axis',(0.,0.,1.));
#10356=DIRECTION('',(-1.,0.,0.));
#10357=DIRECTION('center_axis',(1.,-5.55111512312578E-16,0.));
#10358=DIRECTION('ref_axis',(5.55111512312578E-16,1.,0.));
#10359=DIRECTION('',(1.,0.,0.));
#10360=DIRECTION('center_axis',(0.408248290463862,0.40824829046386,-0.816496580927728));
#10361=DIRECTION('ref_axis',(0.577350269189629,0.577350269189628,0.577350269189621));
#10362=DIRECTION('center_axis',(0.,0.,1.));
#10363=DIRECTION('ref_axis',(1.,0.,0.));
#10364=DIRECTION('center_axis',(1.11022302462516E-16,-1.,0.));
#10365=DIRECTION('ref_axis',(-0.707106781186555,0.,0.70710678118654));
#10366=DIRECTION('center_axis',(0.,-1.,0.));
#10367=DIRECTION('ref_axis',(0.,0.,1.));
#10368=DIRECTION('',(1.11022302462516E-16,-1.,0.));
#10369=DIRECTION('center_axis',(0.,1.,0.));
#10370=DIRECTION('ref_axis',(-1.,0.,0.));
#10371=DIRECTION('',(-1.11022302462516E-16,1.,0.));
#10372=DIRECTION('center_axis',(-0.816496580927725,-0.408248290463869,-0.40824829046386));
#10373=DIRECTION('ref_axis',(-0.577350269189626,0.57735026918963,0.577350269189621));
#10374=DIRECTION('center_axis',(0.,0.,1.));
#10375=DIRECTION('ref_axis',(1.11022302462516E-15,1.,0.));
#10376=DIRECTION('center_axis',(1.,-2.22044604925031E-16,0.));
#10377=DIRECTION('ref_axis',(0.,-0.707106781186555,0.70710678118654));
#10378=DIRECTION('center_axis',(1.,0.,0.));
#10379=DIRECTION('ref_axis',(0.,0.,1.));
#10380=DIRECTION('',(1.,-2.22044604925031E-16,0.));
#10381=DIRECTION('center_axis',(-1.,0.,0.));
#10382=DIRECTION('ref_axis',(0.,-1.,0.));
#10383=DIRECTION('',(-1.,2.22044604925031E-16,0.));
#10384=DIRECTION('center_axis',(-0.816496580927724,0.408248290463871,-0.40824829046386));
#10385=DIRECTION('ref_axis',(-0.577350269189628,-0.577350269189629,0.577350269189621));
#10386=DIRECTION('center_axis',(0.,0.,1.));
#10387=DIRECTION('ref_axis',(-1.,0.,0.));
#10388=DIRECTION('center_axis',(-0.816496580927723,-0.408248290463872,0.408248290463859));
#10389=DIRECTION('ref_axis',(0.577350269189627,-0.577350269189631,0.57735026918962));
#10390=DIRECTION('center_axis',(0.,0.,1.));
#10391=DIRECTION('ref_axis',(5.55111512312576E-16,-1.,0.));
#10392=DIRECTION('center_axis',(0.,0.,1.));
#10393=DIRECTION('ref_axis',(1.,0.,0.));
#10394=DIRECTION('',(0.,0.,1.));
#10395=DIRECTION('center_axis',(0.,0.,1.));
#10396=DIRECTION('ref_axis',(1.,0.,0.));
#10397=DIRECTION('',(0.,0.,1.));
#10398=DIRECTION('center_axis',(1.,0.,0.));
#10399=DIRECTION('ref_axis',(0.,1.,0.));
#10400=DIRECTION('',(0.,0.,1.));
#10401=DIRECTION('',(0.,1.,0.));
#10402=DIRECTION('center_axis',(0.,0.,1.));
#10403=DIRECTION('ref_axis',(5.55111512312576E-16,-1.,0.));
#10404=DIRECTION('',(0.,0.,1.));
#10405=DIRECTION('center_axis',(0.,0.,1.));
#10406=DIRECTION('ref_axis',(5.55111512312576E-16,-1.,0.));
#10407=DIRECTION('center_axis',(-2.22044604925031E-16,-1.,0.));
#10408=DIRECTION('ref_axis',(1.,-2.22044604925031E-16,0.));
#10409=DIRECTION('',(0.,0.,1.));
#10410=DIRECTION('',(1.,-2.22044604925031E-16,0.));
#10411=DIRECTION('center_axis',(0.,0.,1.));
#10412=DIRECTION('ref_axis',(1.,0.,0.));
#10413=DIRECTION('center_axis',(0.,0.,-1.));
#10414=DIRECTION('ref_axis',(1.,0.,0.));
#10415=DIRECTION('center_axis',(0.0398594873598413,-0.995272787934818,-0.0885624009603703));
#10416=DIRECTION('ref_axis',(0.408479397061306,0.0971188838303287,-0.907586086594535));
#10417=DIRECTION('center_axis',(3.52448365596266E-13,1.77635683940025E-13,
-1.));
#10418=DIRECTION('ref_axis',(0.,1.,1.77635683940023E-13));
#10419=DIRECTION('center_axis',(0.892992097097124,0.450072343653862,0.));
#10420=DIRECTION('ref_axis',(-0.450072343653862,0.892992097097124,0.));
#10421=DIRECTION('center_axis',(1.,0.,0.));
#10422=DIRECTION('ref_axis',(0.,0.707106781186487,-0.707106781186609));
#10423=DIRECTION('center_axis',(0.,0.,1.));
#10424=DIRECTION('ref_axis',(0.97288028479796,0.231309211773851,0.));
#10425=DIRECTION('center_axis',(0.,0.,-1.));
#10426=DIRECTION('ref_axis',(0.,1.,0.));
#10427=DIRECTION('',(0.,0.,-1.));
#10428=DIRECTION('',(0.,-1.17758885217183E-15,1.));
#10429=DIRECTION('center_axis',(-0.775565134412812,-0.344096997179426,-0.529240945898311));
#10430=DIRECTION('ref_axis',(0.,0.838378187143696,-0.545088997615665));
#10431=DIRECTION('center_axis',(-0.775565134412822,0.344096997179426,0.529240945898297));
#10432=DIRECTION('ref_axis',(0.,0.838378187143689,-0.545088997615675));
#10433=DIRECTION('center_axis',(0.,-0.843786442012823,0.536679084998978));
#10434=DIRECTION('ref_axis',(0.,0.536679084998978,0.843786442012823));
#10435=DIRECTION('center_axis',(0.,0.838378187143685,-0.545088997615682));
#10436=DIRECTION('ref_axis',(0.,0.545088997615682,0.838378187143685));
#10437=DIRECTION('center_axis',(0.,0.,1.));
#10438=DIRECTION('ref_axis',(0.,1.,0.));
#10439=DIRECTION('center_axis',(0.,0.,-1.));
#10440=DIRECTION('ref_axis',(-0.97288028479796,0.231309211773851,0.));
#10441=DIRECTION('center_axis',(-7.89365027399415E-13,0.,1.));
#10442=DIRECTION('ref_axis',(0.,1.,0.));
#10443=DIRECTION('',(0.,0.,1.));
#10444=DIRECTION('',(0.,1.17758885217183E-15,-1.));
#10445=DIRECTION('center_axis',(-0.0398594873597966,-0.99527278793482,-0.0885624009603697));
#10446=DIRECTION('ref_axis',(-0.408479397061071,0.0971188838302721,-0.907586086594647));
#10447=DIRECTION('center_axis',(-1.,0.,0.));
#10448=DIRECTION('ref_axis',(0.,0.707106781186487,-0.707106781186609));
#10449=DIRECTION('center_axis',(-0.892992097097124,0.450072343653862,0.));
#10450=DIRECTION('ref_axis',(0.450072343653862,0.892992097097124,0.));
#10451=DIRECTION('center_axis',(0.,-1.,-1.17758885217183E-15));
#10452=DIRECTION('ref_axis',(0.,1.17758885217183E-15,-1.));
#10453=DIRECTION('',(1.,0.,0.));
#10454=DIRECTION('',(0.,-1.17758885217183E-15,1.));
#10455=DIRECTION('',(1.,0.,0.));
#10456=DIRECTION('center_axis',(1.,0.,0.));
#10457=DIRECTION('ref_axis',(0.,-0.83837818714366,0.54508899761572));
#10458=DIRECTION('',(-1.,0.,0.));
#10459=DIRECTION('center_axis',(-1.,0.,0.));
#10460=DIRECTION('ref_axis',(0.,-0.958743497277472,0.284272591763895));
#10461=DIRECTION('center_axis',(0.,-0.838378187143685,0.545088997615682));
#10462=DIRECTION('ref_axis',(0.,-0.545088997615682,-0.838378187143685));
#10463=DIRECTION('',(-1.,0.,0.));
#10464=DIRECTION('',(0.,-0.545088997615682,-0.838378187143685));
#10465=DIRECTION('',(1.,0.,0.));
#10466=DIRECTION('',(0.,0.545088997615682,0.838378187143685));
#10467=DIRECTION('center_axis',(1.,0.,0.));
#10468=DIRECTION('ref_axis',(0.,-0.83837818714366,0.54508899761572));
#10469=DIRECTION('',(1.,0.,0.));
#10470=DIRECTION('center_axis',(1.,0.,0.));
#10471=DIRECTION('ref_axis',(0.,-0.958743497277472,0.284272591763895));
#10472=DIRECTION('center_axis',(0.,-1.,-1.17758885217183E-15));
#10473=DIRECTION('ref_axis',(0.,1.17758885217183E-15,-1.));
#10474=DIRECTION('',(1.,0.,0.));
#10475=DIRECTION('',(0.,1.17758885217183E-15,-1.));
#10476=DIRECTION('center_axis',(1.,0.,0.));
#10477=DIRECTION('ref_axis',(0.,0.707106781186493,-0.707106781186602));
#10478=DIRECTION('',(-1.,0.,0.));
#10479=DIRECTION('center_axis',(-1.,0.,0.));
#10480=DIRECTION('ref_axis',(0.,1.,0.));
#10481=DIRECTION('center_axis',(0.,0.,1.));
#10482=DIRECTION('ref_axis',(-1.,-7.55896527404362E-16,0.));
#10483=DIRECTION('center_axis',(0.,0.,1.));
#10484=DIRECTION('ref_axis',(-1.,-1.01064309961486E-15,0.));
#10485=DIRECTION('center_axis',(0.,0.,1.));
#10486=DIRECTION('ref_axis',(-1.,-1.01064309961486E-15,0.));
#10487=DIRECTION('center_axis',(0.892992097097125,-0.450072343653861,0.));
#10488=DIRECTION('ref_axis',(-0.450072343653861,-0.892992097097125,0.));
#10489=DIRECTION('center_axis',(0.,0.,-1.));
#10490=DIRECTION('ref_axis',(-1.,-1.01064309961486E-15,0.));
#10491=DIRECTION('center_axis',(0.0398594873598144,-0.995272787934819,0.0885624009603698));
#10492=DIRECTION('ref_axis',(-0.408479397061211,-0.097118883830298,-0.907586086594581));
#10493=DIRECTION('center_axis',(3.52448365596266E-13,1.77635683940025E-13,
-1.));
#10494=DIRECTION('ref_axis',(0.,-1.,-1.7763568394003E-13));
#10495=DIRECTION('center_axis',(-0.892992097097125,-0.450072343653861,0.));
#10496=DIRECTION('ref_axis',(0.450072343653861,-0.892992097097125,0.));
#10497=DIRECTION('center_axis',(-1.,0.,0.));
#10498=DIRECTION('ref_axis',(0.,-0.707106781186636,-0.707106781186459));
#10499=DIRECTION('center_axis',(0.,0.,1.));
#10500=DIRECTION('ref_axis',(-0.972880284797955,-0.231309211773873,0.));
#10501=DIRECTION('center_axis',(0.,0.,-1.));
#10502=DIRECTION('ref_axis',(0.,-1.,0.));
#10503=DIRECTION('',(0.,0.,-1.));
#10504=DIRECTION('',(0.,1.17758885217183E-15,1.));
#10505=DIRECTION('center_axis',(0.775565134412811,0.344096997179419,-0.529240945898317));
#10506=DIRECTION('ref_axis',(0.,-0.838378187143704,-0.545088997615652));
#10507=DIRECTION('center_axis',(0.775565134412818,-0.344096997179424,0.529240945898304));
#10508=DIRECTION('ref_axis',(-2.77555756156297E-15,-0.838378187143696,-0.545088997615665));
#10509=DIRECTION('center_axis',(0.,0.843786442012823,0.536679084998978));
#10510=DIRECTION('ref_axis',(0.,-0.536679084998978,0.843786442012823));
#10511=DIRECTION('center_axis',(0.,-0.838378187143685,-0.545088997615682));
#10512=DIRECTION('ref_axis',(0.,-0.545088997615682,0.838378187143685));
#10513=DIRECTION('center_axis',(0.,0.,1.));
#10514=DIRECTION('ref_axis',(2.77555756156289E-15,-1.,0.));
#10515=DIRECTION('center_axis',(0.,0.,-1.));
#10516=DIRECTION('ref_axis',(0.97288028479796,-0.231309211773851,0.));
#10517=DIRECTION('center_axis',(0.,0.,1.));
#10518=DIRECTION('ref_axis',(0.,-1.,0.));
#10519=DIRECTION('',(0.,0.,1.));
#10520=DIRECTION('',(0.,-1.17758885217183E-15,-1.));
#10521=DIRECTION('center_axis',(-0.0398594873597704,-0.995272787934834,
0.0885624009602286));
#10522=DIRECTION('ref_axis',(0.408479397060976,-0.0971188838302492,-0.907586086594692));
#10523=DIRECTION('center_axis',(1.,0.,0.));
#10524=DIRECTION('ref_axis',(0.,-0.707106781186636,-0.707106781186459));
#10525=DIRECTION('center_axis',(0.,1.,-1.17758885217183E-15));
#10526=DIRECTION('ref_axis',(0.,1.17758885217183E-15,1.));
#10527=DIRECTION('',(1.,0.,0.));
#10528=DIRECTION('',(0.,1.17758885217183E-15,1.));
#10529=DIRECTION('',(-1.,0.,0.));
#10530=DIRECTION('center_axis',(1.,0.,0.));
#10531=DIRECTION('ref_axis',(0.,1.,-3.55271367880096E-14));
#10532=DIRECTION('',(1.,0.,0.));
#10533=DIRECTION('center_axis',(1.,0.,0.));
#10534=DIRECTION('ref_axis',(0.,0.958743497277472,0.284272591763895));
#10535=DIRECTION('center_axis',(0.,0.838378187143685,0.545088997615682));
#10536=DIRECTION('ref_axis',(0.,-0.545088997615682,0.838378187143685));
#10537=DIRECTION('',(1.,0.,0.));
#10538=DIRECTION('',(0.,0.545088997615682,-0.838378187143685));
#10539=DIRECTION('',(1.,0.,0.));
#10540=DIRECTION('',(0.,-0.545088997615682,0.838378187143685));
#10541=DIRECTION('center_axis',(1.,0.,0.));
#10542=DIRECTION('ref_axis',(0.,1.,-3.55271367880096E-14));
#10543=DIRECTION('',(1.,0.,0.));
#10544=DIRECTION('center_axis',(-1.,0.,0.));
#10545=DIRECTION('ref_axis',(0.,0.958743497277472,0.284272591763895));
#10546=DIRECTION('center_axis',(0.,1.,-1.17758885217183E-15));
#10547=DIRECTION('ref_axis',(0.,1.17758885217183E-15,1.));
#10548=DIRECTION('',(-1.,0.,0.));
#10549=DIRECTION('',(0.,-1.17758885217183E-15,-1.));
#10550=DIRECTION('center_axis',(-1.,0.,0.));
#10551=DIRECTION('ref_axis',(0.,-0.707106781186618,-0.707106781186477));
#10552=DIRECTION('',(1.,0.,0.));
#10553=DIRECTION('center_axis',(1.,0.,0.));
#10554=DIRECTION('ref_axis',(0.,-1.,0.));
#10555=DIRECTION('center_axis',(0.,0.,1.));
#10556=DIRECTION('ref_axis',(1.,0.,0.));
#10557=DIRECTION('center_axis',(0.,0.,-1.));
#10558=DIRECTION('ref_axis',(1.,-8.88178419700125E-16,0.));
#10559=DIRECTION('center_axis',(0.,0.,1.));
#10560=DIRECTION('ref_axis',(1.,-8.88178419700125E-16,0.));
#10561=DIRECTION('center_axis',(1.,0.,0.));
#10562=DIRECTION('ref_axis',(0.,0.707106781186493,-0.707106781186602));
#10563=DIRECTION('center_axis',(-1.,0.,0.));
#10564=DIRECTION('ref_axis',(0.,1.,0.));
#10565=DIRECTION('',(-1.,0.,0.));
#10566=DIRECTION('center_axis',(0.,1.,0.));
#10567=DIRECTION('ref_axis',(1.,0.,0.));
#10568=DIRECTION('center_axis',(0.,0.,1.));
#10569=DIRECTION('ref_axis',(0.707106781186546,0.707106781186549,0.));
#10570=DIRECTION('center_axis',(0.,0.,-1.));
#10571=DIRECTION('ref_axis',(0.707106781186546,0.707106781186549,0.));
#10572=DIRECTION('center_axis',(0.,-1.,0.));
#10573=DIRECTION('ref_axis',(0.707106781186618,0.,-0.707106781186477));
#10574=DIRECTION('center_axis',(5.55111512312578E-15,1.,0.));
#10575=DIRECTION('ref_axis',(1.,-5.55111512312578E-15,0.));
#10576=DIRECTION('',(0.,1.,0.));
#10577=DIRECTION('',(0.,-1.,0.));
#10578=DIRECTION('center_axis',(0.,0.,1.));
#10579=DIRECTION('ref_axis',(0.707106781186546,-0.707106781186549,0.));
#10580=DIRECTION('center_axis',(0.,0.,-1.));
#10581=DIRECTION('ref_axis',(0.707106781186546,-0.707106781186549,0.));
#10582=DIRECTION('center_axis',(0.,-1.17758885217183E-15,1.));
#10583=DIRECTION('ref_axis',(0.707106781186548,0.707106781186548,0.));
#10584=DIRECTION('center_axis',(0.,0.,-1.));
#10585=DIRECTION('ref_axis',(0.,1.,0.));
#10586=DIRECTION('',(0.,1.17758885217183E-15,-1.));
#10587=DIRECTION('center_axis',(0.,0.,1.));
#10588=DIRECTION('ref_axis',(1.,0.,0.));
#10589=DIRECTION('',(0.,0.,-1.));
#10590=DIRECTION('center_axis',(0.,0.,1.));
#10591=DIRECTION('ref_axis',(1.,0.,0.));
#10592=DIRECTION('center_axis',(-1.,0.,0.));
#10593=DIRECTION('ref_axis',(0.,-0.707106781186618,-0.707106781186477));
#10594=DIRECTION('center_axis',(1.,0.,0.));
#10595=DIRECTION('ref_axis',(0.,-1.,0.));
#10596=DIRECTION('',(1.,0.,0.));
#10597=DIRECTION('center_axis',(0.,-1.,0.));
#10598=DIRECTION('ref_axis',(-1.,0.,0.));
#10599=DIRECTION('center_axis',(0.,0.,1.));
#10600=DIRECTION('ref_axis',(-0.707106781186546,-0.707106781186549,0.));
#10601=DIRECTION('center_axis',(0.,0.,-1.));
#10602=DIRECTION('ref_axis',(-0.707106781186546,-0.707106781186549,0.));
#10603=DIRECTION('center_axis',(0.,1.,0.));
#10604=DIRECTION('ref_axis',(-0.707106781186618,0.,-0.707106781186477));
#10605=DIRECTION('center_axis',(5.55111512312578E-15,-1.,0.));
#10606=DIRECTION('ref_axis',(-1.,-5.55111512312578E-15,0.));
#10607=DIRECTION('',(0.,-1.,0.));
#10608=DIRECTION('',(0.,1.,0.));
#10609=DIRECTION('center_axis',(0.,0.,1.));
#10610=DIRECTION('ref_axis',(-0.707106781186546,0.707106781186549,0.));
#10611=DIRECTION('center_axis',(0.,0.,-1.));
#10612=DIRECTION('ref_axis',(-0.707106781186546,0.707106781186549,0.));
#10613=DIRECTION('center_axis',(0.,1.17758885217183E-15,1.));
#10614=DIRECTION('ref_axis',(-0.707106781186548,-0.707106781186548,0.));
#10615=DIRECTION('center_axis',(0.,0.,-1.));
#10616=DIRECTION('ref_axis',(0.,-1.,0.));
#10617=DIRECTION('',(0.,-1.17758885217183E-15,-1.));
#10618=DIRECTION('center_axis',(0.,0.,1.));
#10619=DIRECTION('ref_axis',(1.,0.,0.));
#10620=DIRECTION('center_axis',(0.,0.545088997615682,-0.838378187143685));
#10621=DIRECTION('ref_axis',(0.707106781186562,-0.592822901328176,-0.385436126564212));
#10622=DIRECTION('center_axis',(0.,0.545088997615662,-0.838378187143697));
#10623=DIRECTION('ref_axis',(1.,0.,0.));
#10624=DIRECTION('center_axis',(0.,-0.545088997615661,0.838378187143698));
#10625=DIRECTION('ref_axis',(0.,-0.838378187143698,-0.545088997615661));
#10626=DIRECTION('',(0.,-0.545088997615682,0.838378187143685));
#10627=DIRECTION('center_axis',(-1.,0.,0.));
#10628=DIRECTION('ref_axis',(0.,0.,1.));
#10629=DIRECTION('center_axis',(0.,0.,1.));
#10630=DIRECTION('ref_axis',(0.,-1.,0.));
#10631=DIRECTION('center_axis',(1.,0.,0.));
#10632=DIRECTION('ref_axis',(0.,0.958743497277472,0.284272591763895));
#10633=DIRECTION('center_axis',(0.,-1.17758885217183E-15,-1.));
#10634=DIRECTION('ref_axis',(0.707106781186548,-0.707106781186548,0.));
#10635=DIRECTION('',(0.,1.17758885217183E-15,1.));
#10636=DIRECTION('center_axis',(-2.95822839457884E-27,8.88178419700139E-14,
-1.));
#10637=DIRECTION('ref_axis',(1.,3.33066907387547E-14,0.));
#10638=DIRECTION('center_axis',(1.,0.,0.));
#10639=DIRECTION('ref_axis',(0.,-0.424803640464789,-0.905285516866288));
#10640=DIRECTION('center_axis',(-1.,0.,0.));
#10641=DIRECTION('ref_axis',(0.,-0.424803640464789,-0.905285516866288));
#10642=DIRECTION('center_axis',(1.,0.,0.));
#10643=DIRECTION('ref_axis',(0.,-1.,0.));
#10644=DIRECTION('center_axis',(1.,0.,0.));
#10645=DIRECTION('ref_axis',(0.,-0.958743497277472,0.284272591763895));
#10646=DIRECTION('',(0.,-0.545088997615682,-0.838378187143685));
#10647=DIRECTION('center_axis',(-1.,0.,0.));
#10648=DIRECTION('ref_axis',(0.,0.424803640464811,-0.905285516866278));
#10649=DIRECTION('',(0.,0.,-1.));
#10650=DIRECTION('',(0.,1.,0.));
#10651=DIRECTION('',(0.,0.,-1.));
#10652=DIRECTION('center_axis',(-1.,0.,0.));
#10653=DIRECTION('ref_axis',(0.,1.,0.));
#10654=DIRECTION('',(0.,-1.,0.));
#10655=DIRECTION('center_axis',(-1.,0.,0.));
#10656=DIRECTION('ref_axis',(0.,0.,1.));
#10657=DIRECTION('center_axis',(0.,-0.545088997615734,-0.838378187143651));
#10658=DIRECTION('ref_axis',(0.,0.838378187143651,-0.545088997615734));
#10659=DIRECTION('center_axis',(0.,0.545088997615682,0.838378187143685));
#10660=DIRECTION('ref_axis',(0.707106781186561,0.592822901328178,-0.385436126564211));
#10661=DIRECTION('center_axis',(0.,-0.545088997615661,-0.838378187143698));
#10662=DIRECTION('ref_axis',(0.,0.838378187143698,-0.545088997615661));
#10663=DIRECTION('center_axis',(0.,0.,-1.));
#10664=DIRECTION('ref_axis',(5.55111512312587E-15,1.,0.));
#10665=DIRECTION('center_axis',(1.,0.,0.));
#10666=DIRECTION('ref_axis',(0.,0.424803640464811,-0.905285516866278));
#10667=DIRECTION('center_axis',(0.,-0.545088997615682,-0.838378187143685));
#10668=DIRECTION('ref_axis',(-0.707106781186561,0.592822901328178,-0.385436126564211));
#10669=DIRECTION('center_axis',(0.,-0.545088997615662,-0.838378187143697));
#10670=DIRECTION('ref_axis',(-1.,0.,0.));
#10671=DIRECTION('center_axis',(0.,0.545088997615662,0.838378187143697));
#10672=DIRECTION('ref_axis',(0.,0.838378187143697,-0.545088997615662));
#10673=DIRECTION('',(0.,0.545088997615682,0.838378187143685));
#10674=DIRECTION('center_axis',(1.,0.,0.));
#10675=DIRECTION('ref_axis',(0.,0.,-1.));
#10676=DIRECTION('center_axis',(0.,0.,1.));
#10677=DIRECTION('ref_axis',(0.,1.,0.));
#10678=DIRECTION('center_axis',(-1.,0.,0.));
#10679=DIRECTION('ref_axis',(0.,-0.958743497277472,0.284272591763895));
#10680=DIRECTION('center_axis',(0.,1.17758885217183E-15,-1.));
#10681=DIRECTION('ref_axis',(-0.707106781186548,0.707106781186548,0.));
#10682=DIRECTION('',(0.,-1.17758885217183E-15,1.));
#10683=DIRECTION('center_axis',(0.,0.,-1.));
#10684=DIRECTION('ref_axis',(-1.,-2.22044604925031E-14,0.));
#10685=DIRECTION('center_axis',(-1.,0.,0.));
#10686=DIRECTION('ref_axis',(0.,0.424803640464792,-0.905285516866286));
#10687=DIRECTION('center_axis',(1.,0.,0.));
#10688=DIRECTION('ref_axis',(0.,0.424803640464792,-0.905285516866286));
#10689=DIRECTION('center_axis',(-1.,0.,0.));
#10690=DIRECTION('ref_axis',(0.,1.,0.));
#10691=DIRECTION('center_axis',(-1.,0.,0.));
#10692=DIRECTION('ref_axis',(0.,0.958743497277472,0.284272591763895));
#10693=DIRECTION('',(0.,0.545088997615682,-0.838378187143685));
#10694=DIRECTION('center_axis',(1.,0.,0.));
#10695=DIRECTION('ref_axis',(0.,-0.424803640464792,-0.905285516866286));
#10696=DIRECTION('',(0.,0.,-1.));
#10697=DIRECTION('',(0.,-1.,0.));
#10698=DIRECTION('',(0.,0.,-1.));
#10699=DIRECTION('',(0.,1.,0.));
#10700=DIRECTION('center_axis',(1.,0.,0.));
#10701=DIRECTION('ref_axis',(0.,1.,0.));
#10702=DIRECTION('center_axis',(1.,0.,0.));
#10703=DIRECTION('ref_axis',(0.,0.,-1.));
#10704=DIRECTION('center_axis',(0.,0.545088997615732,-0.838378187143652));
#10705=DIRECTION('ref_axis',(0.,-0.838378187143652,-0.545088997615732));
#10706=DIRECTION('center_axis',(0.,-0.545088997615682,0.838378187143685));
#10707=DIRECTION('ref_axis',(-0.707106781186561,-0.592822901328178,-0.385436126564211));
#10708=DIRECTION('center_axis',(0.,0.545088997615661,-0.838378187143698));
#10709=DIRECTION('ref_axis',(0.,-0.838378187143698,-0.545088997615661));
#10710=DIRECTION('center_axis',(-8.88178419700124E-14,0.,-1.));
#10711=DIRECTION('ref_axis',(0.,-1.,0.));
#10712=DIRECTION('center_axis',(-1.,0.,0.));
#10713=DIRECTION('ref_axis',(0.,-0.424803640464792,-0.905285516866286));
#10714=DIRECTION('center_axis',(1.,0.,0.));
#10715=DIRECTION('ref_axis',(0.,0.838378187143673,-0.545088997615699));
#10716=DIRECTION('',(-1.,0.,0.));
#10717=DIRECTION('center_axis',(1.,0.,0.));
#10718=DIRECTION('ref_axis',(0.,-1.,-4.4408920985003E-14));
#10719=DIRECTION('',(-1.,0.,0.));
#10720=DIRECTION('center_axis',(0.,1.,0.));
#10721=DIRECTION('ref_axis',(1.,0.,0.));
#10722=DIRECTION('',(0.,0.,-1.));
#10723=DIRECTION('',(-1.,0.,0.));
#10724=DIRECTION('',(0.,0.,-1.));
#10725=DIRECTION('center_axis',(-1.11022302462516E-16,-1.,0.));
#10726=DIRECTION('ref_axis',(-1.,1.11022302462516E-16,0.));
#10727=DIRECTION('',(0.,0.,-1.));
#10728=DIRECTION('',(1.,-1.11022302462516E-16,0.));
#10729=DIRECTION('',(0.,0.,-1.));
#10730=DIRECTION('center_axis',(1.,0.,0.));
#10731=DIRECTION('ref_axis',(0.,-8.26946079742758E-16,1.));
#10732=DIRECTION('',(1.,0.,0.));
#10733=DIRECTION('center_axis',(1.,0.,0.));
#10734=DIRECTION('ref_axis',(0.,1.,0.));
#10735=DIRECTION('',(-1.,0.,0.));
#10736=DIRECTION('center_axis',(0.,0.,-1.));
#10737=DIRECTION('ref_axis',(0.,1.,0.));
#10738=DIRECTION('',(0.,1.,0.));
#10739=DIRECTION('center_axis',(1.,0.,0.));
#10740=DIRECTION('ref_axis',(0.,1.,0.));
#10741=DIRECTION('center_axis',(0.,0.,-1.));
#10742=DIRECTION('ref_axis',(0.,1.,0.));
#10743=DIRECTION('',(1.,0.,0.));
#10744=DIRECTION('',(0.,-1.,0.));
#10745=DIRECTION('',(-1.,0.,0.));
#10746=DIRECTION('center_axis',(1.,0.,0.));
#10747=DIRECTION('ref_axis',(0.,1.,0.));
#10748=DIRECTION('center_axis',(-1.,0.,0.));
#10749=DIRECTION('ref_axis',(0.,1.,0.));
#10750=DIRECTION('center_axis',(1.,0.,0.));
#10751=DIRECTION('ref_axis',(0.,-8.26946079742758E-16,1.));
#10752=DIRECTION('center_axis',(0.,0.,-1.));
#10753=DIRECTION('ref_axis',(0.,1.,0.));
#10754=DIRECTION('center_axis',(0.,0.,1.));
#10755=DIRECTION('ref_axis',(0.,1.,0.));
#10756=DIRECTION('center_axis',(0.,0.,-1.));
#10757=DIRECTION('ref_axis',(-1.,-5.55111512312578E-15,0.));
#10758=DIRECTION('center_axis',(0.,0.,1.));
#10759=DIRECTION('ref_axis',(-1.,-5.55111512312578E-15,0.));
#10760=DIRECTION('center_axis',(0.,0.,-1.));
#10761=DIRECTION('ref_axis',(2.77555756156287E-15,-1.,0.));
#10762=DIRECTION('center_axis',(0.,0.,1.));
#10763=DIRECTION('ref_axis',(2.77555756156287E-15,-1.,0.));
#10764=DIRECTION('center_axis',(0.,0.,-1.));
#10765=DIRECTION('ref_axis',(1.,5.55111512312578E-15,0.));
#10766=DIRECTION('center_axis',(0.,0.,1.));
#10767=DIRECTION('ref_axis',(1.,5.55111512312578E-15,0.));
#10768=DIRECTION('center_axis',(0.,0.,1.));
#10769=DIRECTION('ref_axis',(-1.,0.,0.));
#10770=DIRECTION('',(0.,0.,1.));
#10771=DIRECTION('center_axis',(0.,0.,1.));
#10772=DIRECTION('ref_axis',(-1.,0.,0.));
#10773=DIRECTION('center_axis',(-1.,-1.11022302462516E-16,0.));
#10774=DIRECTION('ref_axis',(1.11022302462516E-16,-1.,0.));
#10775=DIRECTION('',(0.,0.,1.));
#10776=DIRECTION('',(1.11022302462516E-16,-1.,0.));
#10777=DIRECTION('center_axis',(0.,0.,1.));
#10778=DIRECTION('ref_axis',(1.11022302462516E-15,1.,0.));
#10779=DIRECTION('',(0.,0.,1.));
#10780=DIRECTION('center_axis',(0.,0.,1.));
#10781=DIRECTION('ref_axis',(1.11022302462516E-15,1.,0.));
#10782=DIRECTION('center_axis',(0.,1.,0.));
#10783=DIRECTION('ref_axis',(-1.,0.,0.));
#10784=DIRECTION('',(-1.,0.,0.));
#10785=DIRECTION('center_axis',(0.,0.,1.));
#10786=DIRECTION('ref_axis',(1.,0.,0.));
#12957=CARTESIAN_POINT('',(0.,0.,0.));
#12958=CARTESIAN_POINT('Origin',(3.5,1.43177298256785,258.886209595194));
#12959=CARTESIAN_POINT('',(3.5,-3.56822701743216,260.886209595194));
#12960=CARTESIAN_POINT('',(5.5,-3.56822701743215,258.886209595194));
#12961=CARTESIAN_POINT('Origin',(3.5,-3.56822701743215,258.886209595194));
#12962=CARTESIAN_POINT('',(5.5,16.4317729825678,258.886209595194));
#12963=CARTESIAN_POINT('',(5.5,1.43177298256785,258.886209595194));
#12964=CARTESIAN_POINT('',(3.5,16.4317729825678,260.886209595194));
#12965=CARTESIAN_POINT('Origin',(3.5,16.4317729825678,258.886209595194));
#12966=CARTESIAN_POINT('',(3.5,1.43177298256785,260.886209595194));
#12967=CARTESIAN_POINT('Origin',(-1.5,16.4317729825679,258.886209595194));
#12968=CARTESIAN_POINT('',(3.5,18.4317729825679,258.886209595194));
#12969=CARTESIAN_POINT('Origin',(3.5,16.4317729825679,258.886209595194));
#12970=CARTESIAN_POINT('',(-16.5,18.4317729825679,258.886209595194));
#12971=CARTESIAN_POINT('',(-1.5,18.4317729825679,258.886209595194));
#12972=CARTESIAN_POINT('',(-16.5,16.4317729825679,260.886209595194));
#12973=CARTESIAN_POINT('Origin',(-16.5,16.4317729825679,258.886209595194));
#12974=CARTESIAN_POINT('',(-1.5,16.4317729825679,260.886209595194));
#12975=CARTESIAN_POINT('Origin',(3.5,16.4317729825678,258.886209595194));
#12976=CARTESIAN_POINT('Origin',(3.5,16.4317729825678,258.886209595194));
#12977=CARTESIAN_POINT('Origin',(-16.5,11.4317729825679,258.886209595194));
#12978=CARTESIAN_POINT('',(-18.5,16.4317729825679,258.886209595194));
#12979=CARTESIAN_POINT('Origin',(-16.5,16.4317729825679,258.886209595194));
#12980=CARTESIAN_POINT('',(-18.5,-3.56822701743215,258.886209595194));
#12981=CARTESIAN_POINT('',(-18.5,11.4317729825679,258.886209595194));
#12982=CARTESIAN_POINT('',(-16.5,-3.56822701743215,260.886209595194));
#12983=CARTESIAN_POINT('Origin',(-16.5,-3.56822701743215,258.886209595194));
#12984=CARTESIAN_POINT('',(-16.5,11.4317729825679,260.886209595194));
#12985=CARTESIAN_POINT('Origin',(-16.5,16.4317729825679,258.886209595194));
#12986=CARTESIAN_POINT('Origin',(-16.5,16.4317729825679,258.886209595194));
#12987=CARTESIAN_POINT('Origin',(-11.5,-3.56822701743215,258.886209595194));
#12988=CARTESIAN_POINT('',(-16.5,-5.56822701743215,258.886209595194));
#12989=CARTESIAN_POINT('Origin',(-16.5,-3.56822701743215,258.886209595194));
#12990=CARTESIAN_POINT('',(3.5,-5.56822701743215,258.886209595194));
#12991=CARTESIAN_POINT('',(-11.5,-5.56822701743215,258.886209595194));
#12992=CARTESIAN_POINT('Origin',(3.5,-3.56822701743216,258.886209595194));
#12993=CARTESIAN_POINT('',(-11.5,-3.56822701743215,260.886209595194));
#12994=CARTESIAN_POINT('Origin',(-16.5,-3.56822701743215,258.886209595194));
#12995=CARTESIAN_POINT('Origin',(-16.5,-3.56822701743215,258.886209595194));
#12996=CARTESIAN_POINT('Origin',(3.5,-3.56822701743215,258.886209595194));
#12997=CARTESIAN_POINT('Origin',(3.5,-3.56822701743215,258.886209595194));
#12998=CARTESIAN_POINT('Origin',(3.5,16.4317729825678,256.886209595194));
#12999=CARTESIAN_POINT('',(5.5,16.4317729825678,256.886209595194));
#13000=CARTESIAN_POINT('',(5.5,16.4317729825678,256.886209595194));
#13001=CARTESIAN_POINT('',(3.5,18.4317729825679,256.886209595194));
#13002=CARTESIAN_POINT('Origin',(3.5,16.4317729825678,256.886209595194));
#13003=CARTESIAN_POINT('',(3.5,18.4317729825679,256.886209595194));
#13004=CARTESIAN_POINT('Origin',(5.5,-3.56822701743215,256.886209595194));
#13005=CARTESIAN_POINT('',(5.5,-3.56822701743215,256.886209595194));
#13006=CARTESIAN_POINT('',(5.5,-3.56822701743215,256.886209595194));
#13007=CARTESIAN_POINT('',(5.5,-3.56822701743215,256.886209595194));
#13008=CARTESIAN_POINT('Origin',(3.5,-3.56822701743215,256.886209595194));
#13009=CARTESIAN_POINT('',(3.5,-5.56822701743215,256.886209595194));
#13010=CARTESIAN_POINT('',(3.5,-5.56822701743215,256.886209595194));
#13011=CARTESIAN_POINT('Origin',(3.5,-3.56822701743215,256.886209595194));
#13012=CARTESIAN_POINT('Origin',(-16.5,-5.56822701743215,256.886209595194));
#13013=CARTESIAN_POINT('',(-16.5,-5.56822701743215,256.886209595194));
#13014=CARTESIAN_POINT('',(-16.5,-5.56822701743215,256.886209595194));
#13015=CARTESIAN_POINT('',(-16.5,-5.56822701743215,256.886209595194));
#13016=CARTESIAN_POINT('Origin',(-6.5,6.43177298256785,260.886209595194));
#13017=CARTESIAN_POINT('',(-15.5,6.43177298256785,260.886209595194));
#13018=CARTESIAN_POINT('Origin',(-6.5,6.43177298256785,260.886209595194));
#13019=CARTESIAN_POINT('Origin',(-10.6406655616155,14.6473002758614,247.086209595194));
#13020=CARTESIAN_POINT('',(-10.6406655616155,14.8473002758614,247.086209595194));
#13021=CARTESIAN_POINT('',(-10.5506510928848,14.468701856442,247.086209595194));
#13022=CARTESIAN_POINT('Origin',(-10.6406655616155,14.6473002758614,247.086209595194));
#13023=CARTESIAN_POINT('',(-10.6406655616155,14.6473002758614,246.886209595194));
#13024=CARTESIAN_POINT('Origin',(-10.6406655616155,14.6473002758614,247.086209595194));
#13025=CARTESIAN_POINT('Origin',(-10.6406655616155,14.6473002758614,247.086209595194));
#13026=CARTESIAN_POINT('Origin',(-10.6406655616156,14.6473002758614,256.886209595194));
#13027=CARTESIAN_POINT('',(-10.6406655616156,14.8473002758614,250.657383286513));
#13028=CARTESIAN_POINT('',(-10.5506510928848,14.468701856442,250.657383286513));
#13029=CARTESIAN_POINT('Origin',(-10.6406655616156,14.6473002758614,250.657383286513));
#13030=CARTESIAN_POINT('',(-10.5506510928848,14.468701856442,256.886209595194));
#13031=CARTESIAN_POINT('',(-10.6406655616156,14.8473002758614,256.886209595194));
#13032=CARTESIAN_POINT('Ctrl Pts',(-10.6406655616155,14.8473002758614,250.657383286513));
#13033=CARTESIAN_POINT('Ctrl Pts',(-10.6406655616155,14.8473002758614,250.772822299168));
#13034=CARTESIAN_POINT('Ctrl Pts',(-10.538120734944,14.8908595770985,250.995273591613));
#13035=CARTESIAN_POINT('Ctrl Pts',(-10.3384894997035,14.9691998711056,251.141377231877));
#13036=CARTESIAN_POINT('Ctrl Pts',(-10.2310529316636,15.0089220887177,251.202472284128));
#13037=CARTESIAN_POINT('Ctrl Pts',(-10.5897180129765,14.8473002758614,250.657383286513));
#13038=CARTESIAN_POINT('Ctrl Pts',(-10.5897180129765,14.8473002758614,250.761141960988));
#13039=CARTESIAN_POINT('Ctrl Pts',(-10.4974067252999,14.881909580796,250.965068827275));
#13040=CARTESIAN_POINT('Ctrl Pts',(-10.305922542976,14.9524957418658,251.110832462786));
#13041=CARTESIAN_POINT('Ctrl Pts',(-10.2016668934649,14.9892426247285,251.172204138164));
#13042=CARTESIAN_POINT('Ctrl Pts',(-10.4881554517255,14.8062503675603,250.657383286512));
#13043=CARTESIAN_POINT('Ctrl Pts',(-10.4881554517255,14.8062503675603,250.742595721283));
#13044=CARTESIAN_POINT('Ctrl Pts',(-10.4162137192475,14.8272257027818,250.918324937551));
#13045=CARTESIAN_POINT('Ctrl Pts',(-10.2409200923139,14.8880763812795,251.067105998786));
#13046=CARTESIAN_POINT('Ctrl Pts',(-10.1430306190524,14.921491757668,251.130326463532));
#13047=CARTESIAN_POINT('Ctrl Pts',(-10.4201854941467,14.6565138525604,250.657383286513));
#13048=CARTESIAN_POINT('Ctrl Pts',(-10.4201854941467,14.6565138525604,250.744356284269));
#13049=CARTESIAN_POINT('Ctrl Pts',(-10.3574107201025,14.6791700163663,250.925879494604));
#13050=CARTESIAN_POINT('Ctrl Pts',(-10.190502594735,14.7458320313741,251.084602237115));
#13051=CARTESIAN_POINT('Ctrl Pts',(-10.0960822918466,14.782338215616,251.152000580692));
#13052=CARTESIAN_POINT('Ctrl Pts',(-10.4659883159327,14.5274464330055,250.657383286513));
#13053=CARTESIAN_POINT('Ctrl Pts',(-10.4659883159327,14.5274464330055,250.769730689183));
#13054=CARTESIAN_POINT('Ctrl Pts',(-10.3869339431387,14.5654984247408,250.993661589234));
#13055=CARTESIAN_POINT('Ctrl Pts',(-10.2083950877898,14.6468617222379,251.161662391349));
#13056=CARTESIAN_POINT('Ctrl Pts',(-10.1097392710433,14.6894222004357,251.232425194565));
#13057=CARTESIAN_POINT('Ctrl Pts',(-10.5279032137342,14.4801668977517,250.657383286513));
#13058=CARTESIAN_POINT('Ctrl Pts',(-10.5279032137342,14.4801668977517,250.789388896832));
#13059=CARTESIAN_POINT('Ctrl Pts',(-10.4330225721765,14.5282019689485,251.045597317344));
#13060=CARTESIAN_POINT('Ctrl Pts',(-10.2421023786097,14.6177277546944,251.219068720891));
#13061=CARTESIAN_POINT('Ctrl Pts',(-10.138683251246,14.6634274904892,251.291741549006));
#13062=CARTESIAN_POINT('Ctrl Pts',(-10.5506510928848,14.468701856442,250.657383286513));
#13063=CARTESIAN_POINT('Ctrl Pts',(-10.5506510928848,14.468701856442,250.795910101699));
#13064=CARTESIAN_POINT('Ctrl Pts',(-10.4503355015756,14.519836688329,251.062851652633));
#13065=CARTESIAN_POINT('Ctrl Pts',(-10.2550440757969,14.6118013812939,251.23817602095));
#13066=CARTESIAN_POINT('Ctrl Pts',(-10.1499430853231,14.6584318106646,251.311490083651));
#13067=CARTESIAN_POINT('',(-10.2310529316636,15.0089220887177,251.202472284128));
#13068=CARTESIAN_POINT('',(-10.1499430853231,14.6584318106646,251.311490083651));
#13069=CARTESIAN_POINT('Origin',(-10.2310529316636,14.841246451289,251.311490083651));
#13070=CARTESIAN_POINT('Ctrl Pts',(-10.1499430853231,14.6584318106646,251.311490083651));
#13071=CARTESIAN_POINT('Ctrl Pts',(-10.2550440757969,14.6118013812939,251.23817602095));
#13072=CARTESIAN_POINT('Ctrl Pts',(-10.4503355015756,14.519836688329,251.062851652633));
#13073=CARTESIAN_POINT('Ctrl Pts',(-10.5506510928848,14.468701856442,250.795910101699));
#13074=CARTESIAN_POINT('Ctrl Pts',(-10.5506510928848,14.468701856442,250.657383286513));
#13075=CARTESIAN_POINT('Ctrl Pts',(-10.6406655616155,14.8473002758614,250.657383286513));
#13076=CARTESIAN_POINT('Ctrl Pts',(-10.6406655616155,14.8473002758614,250.772822299168));
#13077=CARTESIAN_POINT('Ctrl Pts',(-10.538120734944,14.8908595770985,250.995273591613));
#13078=CARTESIAN_POINT('Ctrl Pts',(-10.3384894997035,14.9691998711056,251.141377231877));
#13079=CARTESIAN_POINT('Ctrl Pts',(-10.2310529316636,15.0089220887177,251.202472284128));
#13080=CARTESIAN_POINT('Ctrl Pts',(-10.2310529316636,15.0089220887177,251.202472284128));
#13081=CARTESIAN_POINT('Ctrl Pts',(-9.22773159688035,15.4540682707548,251.887132680399));
#13082=CARTESIAN_POINT('Ctrl Pts',(-7.42162795596114,15.8927893964761,252.561910971013));
#13083=CARTESIAN_POINT('Ctrl Pts',(-4.84661911018312,15.73844540057,252.324521040102));
#13084=CARTESIAN_POINT('Ctrl Pts',(-3.43782795819191,15.3056862100758,251.658912548309));
#13085=CARTESIAN_POINT('Ctrl Pts',(-2.76894706833641,15.0089220887177,251.202472284128));
#13086=CARTESIAN_POINT('Ctrl Pts',(-10.2016668934649,14.9892426247285,251.172204138164));
#13087=CARTESIAN_POINT('Ctrl Pts',(-9.20327283417141,15.431382290481,251.852198827549));
#13088=CARTESIAN_POINT('Ctrl Pts',(-7.41197152048377,15.8650501229424,252.519151822071));
#13089=CARTESIAN_POINT('Ctrl Pts',(-4.8634067476038,15.7126700064094,252.284802719314));
#13090=CARTESIAN_POINT('Ctrl Pts',(-3.46392914606411,15.2840024018968,251.625533931087));
#13091=CARTESIAN_POINT('Ctrl Pts',(-2.79833310653512,14.9892426247285,251.172204138164));
#13092=CARTESIAN_POINT('Ctrl Pts',(-10.1430306190534,14.9214917576807,251.130326463525));
#13093=CARTESIAN_POINT('Ctrl Pts',(-9.15449162417327,15.3560276990127,251.802015417513));
#13094=CARTESIAN_POINT('Ctrl Pts',(-7.39262374638816,15.7776019247494,252.454602616968));
#13095=CARTESIAN_POINT('Ctrl Pts',(-4.89695559334381,15.6298815734355,252.225862811528));
#13096=CARTESIAN_POINT('Ctrl Pts',(-3.51599537753336,15.2111823852354,251.578119099517));
#13097=CARTESIAN_POINT('Ctrl Pts',(-2.85696938094662,14.9214917576808,251.130326463525));
#13098=CARTESIAN_POINT('Ctrl Pts',(-10.0960822918478,14.7823382156223,251.152000580689));
#13099=CARTESIAN_POINT('Ctrl Pts',(-9.11745075691728,15.2086150138118,251.821482469268));
#13100=CARTESIAN_POINT('Ctrl Pts',(-7.37894869396555,15.6193010674826,252.469869887398));
#13101=CARTESIAN_POINT('Ctrl Pts',(-4.92106363262171,15.4756382751295,252.242792745249));
#13102=CARTESIAN_POINT('Ctrl Pts',(-3.55633873143921,15.0665227477487,251.598321839742));
#13103=CARTESIAN_POINT('Ctrl Pts',(-2.90391770815218,14.7823382156223,251.152000580689));
#13104=CARTESIAN_POINT('Ctrl Pts',(-10.1097392710443,14.689422200441,251.232425194563));
#13105=CARTESIAN_POINT('Ctrl Pts',(-9.13234066037412,15.1172900370079,251.909075130909));
#13106=CARTESIAN_POINT('Ctrl Pts',(-7.38629562289862,15.5332576390045,252.569858388844));
#13107=CARTESIAN_POINT('Ctrl Pts',(-4.90876172522952,15.3874061283022,252.337941576935));
#13108=CARTESIAN_POINT('Ctrl Pts',(-3.54185980273583,14.9746674248189,251.683525152127));
#13109=CARTESIAN_POINT('Ctrl Pts',(-2.89026072895573,14.689422200441,251.232425194563));
#13110=CARTESIAN_POINT('Ctrl Pts',(-10.138683251246,14.6634274904892,251.291741549006));
#13111=CARTESIAN_POINT('Ctrl Pts',(-9.15845858332119,15.0967361952484,251.97440989295));
#13112=CARTESIAN_POINT('Ctrl Pts',(-7.39747124224787,15.5223048250492,252.645709370518));
#13113=CARTESIAN_POINT('Ctrl Pts',(-4.8896809061876,15.3727131232182,252.409679681977));
#13114=CARTESIAN_POINT('Ctrl Pts',(-3.51479986070389,14.9522999603287,251.746853778302));
#13115=CARTESIAN_POINT('Ctrl Pts',(-2.86131674875402,14.6634274904892,251.291741549006));
#13116=CARTESIAN_POINT('Ctrl Pts',(-10.1499430853231,14.6584318106646,251.311490083651));
#13117=CARTESIAN_POINT('Ctrl Pts',(-9.16843308390469,15.0939009017879,251.996150479922));
#13118=CARTESIAN_POINT('Ctrl Pts',(-7.40159256561416,15.5230846117326,252.670928770536));
#13119=CARTESIAN_POINT('Ctrl Pts',(-4.88256217300522,15.3720959200853,252.433538839625));
#13120=CARTESIAN_POINT('Ctrl Pts',(-3.50439691562252,14.9487445380801,251.767930347832));
#13121=CARTESIAN_POINT('Ctrl Pts',(-2.85005691467692,14.6584318106646,251.311490083651));
#13122=CARTESIAN_POINT('',(-2.76894706833642,15.0089220887177,251.202472284128));
#13123=CARTESIAN_POINT('',(-2.85005691467693,14.6584318106646,251.311490083651));
#13124=CARTESIAN_POINT('Origin',(-2.76894706833642,14.841246451289,251.311490083651));
#13125=CARTESIAN_POINT('Origin',(-6.5,6.43177298256785,238.377236865592));
#13126=CARTESIAN_POINT('Origin',(-6.5,6.59944861999658,238.268219066069));
#13127=CARTESIAN_POINT('Ctrl Pts',(-2.7689470683364,15.0089220887177,251.202472284128));
#13128=CARTESIAN_POINT('Ctrl Pts',(-2.66150284572828,14.9691970410038,251.141372879018));
#13129=CARTESIAN_POINT('Ctrl Pts',(-2.46188597582478,14.8908631544399,250.995305022995));
#13130=CARTESIAN_POINT('Ctrl Pts',(-2.35933443838445,14.8473002758614,250.772830523889));
#13131=CARTESIAN_POINT('Ctrl Pts',(-2.35933443838446,14.8473002758614,250.657383286513));
#13132=CARTESIAN_POINT('Ctrl Pts',(-2.7983331065351,14.9892426247285,251.172204138164));
#13133=CARTESIAN_POINT('Ctrl Pts',(-2.69407002908775,14.9524931237486,251.110828090218));
#13134=CARTESIAN_POINT('Ctrl Pts',(-2.50259872954677,14.8819120216761,250.965097541818));
#13135=CARTESIAN_POINT('Ctrl Pts',(-2.41028198702348,14.8473002758614,250.761149353516));
#13136=CARTESIAN_POINT('Ctrl Pts',(-2.41028198702349,14.8473002758614,250.657383286513));
#13137=CARTESIAN_POINT('Ctrl Pts',(-2.85696936415237,14.9214919773635,251.130326345305));
#13138=CARTESIAN_POINT('Ctrl Pts',(-2.75907291652762,14.8880742202187,251.067101376269));
#13139=CARTESIAN_POINT('Ctrl Pts',(-2.58378919283628,14.8272266541689,250.91834948267));
#13140=CARTESIAN_POINT('Ctrl Pts',(-2.51184450813729,14.8062507365839,250.742601792441));
#13141=CARTESIAN_POINT('Ctrl Pts',(-2.5118445081373,14.8062507365839,250.657383286513));
#13142=CARTESIAN_POINT('Ctrl Pts',(-2.90391768707942,14.7823383248995,251.152000540521));
#13143=CARTESIAN_POINT('Ctrl Pts',(-2.80949065699697,14.7458295396896,251.084597394993));
#13144=CARTESIAN_POINT('Ctrl Pts',(-2.64259110444924,14.6791708676688,250.92590490699));
#13145=CARTESIAN_POINT('Ctrl Pts',(-2.5798144560163,14.6565140249316,250.744362480863));
#13146=CARTESIAN_POINT('Ctrl Pts',(-2.57981445601631,14.6565140249316,250.657383286513));
#13147=CARTESIAN_POINT('Ctrl Pts',(-2.89026071151903,14.6894222918615,251.232425160676));
#13148=CARTESIAN_POINT('Ctrl Pts',(-2.79159786580937,14.6468587813434,251.161657315799));
#13149=CARTESIAN_POINT('Ctrl Pts',(-2.613069944193,14.5655011103562,250.993693104898));
#13150=CARTESIAN_POINT('Ctrl Pts',(-2.53401164238394,14.5274465772739,250.769738693635));
#13151=CARTESIAN_POINT('Ctrl Pts',(-2.53401164238394,14.5274465772739,250.657383286513));
#13152=CARTESIAN_POINT('Ctrl Pts',(-2.861316748754,14.6634274904892,251.291741549006));
#13153=CARTESIAN_POINT('Ctrl Pts',(-2.75789025305402,14.6177244987105,251.219063543146));
#13154=CARTESIAN_POINT('Ctrl Pts',(-2.56698332287745,14.5282057767213,251.045633492924));
#13155=CARTESIAN_POINT('Ctrl Pts',(-2.47209678626579,14.4801668977517,250.789398301879));
#13156=CARTESIAN_POINT('Ctrl Pts',(-2.4720967862658,14.4801668977517,250.657383286513));
#13157=CARTESIAN_POINT('Ctrl Pts',(-2.8500569146769,14.6584318106646,251.311490083651));
#13158=CARTESIAN_POINT('Ctrl Pts',(-2.74494843603853,14.6117980590005,251.238170797519));
#13159=CARTESIAN_POINT('Ctrl Pts',(-2.54967106330685,14.5198408878167,251.062889370291));
#13160=CARTESIAN_POINT('Ctrl Pts',(-2.44934890711523,14.468701856442,250.795919971364));
#13161=CARTESIAN_POINT('Ctrl Pts',(-2.44934890711523,14.468701856442,250.657383286513));
#13162=CARTESIAN_POINT('',(-2.35933443838446,14.8473002758614,250.657383286513));
#13163=CARTESIAN_POINT('',(-2.44934890711523,14.468701856442,250.657383286513));
#13164=CARTESIAN_POINT('Origin',(-2.35933443838446,14.6473002758614,250.657383286513));
#13165=CARTESIAN_POINT('Ctrl Pts',(-2.44934890711523,14.468701856442,250.657383286513));
#13166=CARTESIAN_POINT('Ctrl Pts',(-2.44934890711523,14.468701856442,250.795919971364));
#13167=CARTESIAN_POINT('Ctrl Pts',(-2.54967106330685,14.5198408878167,251.062889370291));
#13168=CARTESIAN_POINT('Ctrl Pts',(-2.74494843603853,14.6117980590005,251.238170797519));
#13169=CARTESIAN_POINT('Ctrl Pts',(-2.8500569146769,14.6584318106646,251.311490083651));
#13170=CARTESIAN_POINT('Ctrl Pts',(-2.7689470683364,15.0089220887177,251.202472284128));
#13171=CARTESIAN_POINT('Ctrl Pts',(-2.66150284572828,14.9691970410038,251.141372879018));
#13172=CARTESIAN_POINT('Ctrl Pts',(-2.46188597582478,14.8908631544399,250.995305022995));
#13173=CARTESIAN_POINT('Ctrl Pts',(-2.35933443838445,14.8473002758614,250.772830523889));
#13174=CARTESIAN_POINT('Ctrl Pts',(-2.35933443838446,14.8473002758614,250.657383286513));
#13175=CARTESIAN_POINT('Origin',(-2.35933443838445,14.6473002758614,256.886209595194));
#13176=CARTESIAN_POINT('',(-2.35933443838445,14.8473002758614,247.086209595194));
#13177=CARTESIAN_POINT('',(-2.44934890711522,14.468701856442,247.086209595194));
#13178=CARTESIAN_POINT('Origin',(-2.35933443838445,14.6473002758614,247.086209595194));
#13179=CARTESIAN_POINT('',(-2.44934890711522,14.468701856442,256.886209595194));
#13180=CARTESIAN_POINT('',(-2.35933443838445,14.8473002758614,256.886209595194));
#13181=CARTESIAN_POINT('Origin',(-2.35933443838447,14.6473002758614,247.086209595194));
#13182=CARTESIAN_POINT('',(-2.35933443838447,14.6473002758614,246.886209595194));
#13183=CARTESIAN_POINT('Origin',(-2.35933443838447,14.6473002758614,247.086209595194));
#13184=CARTESIAN_POINT('Origin',(-2.35933443838447,14.6473002758614,247.086209595194));
#13185=CARTESIAN_POINT('Origin',(-6.5,14.8473002758614,250.657383286513));
#13186=CARTESIAN_POINT('',(3.5,14.8473002758614,250.657383286513));
#13187=CARTESIAN_POINT('',(-6.5,14.8473002758614,250.657383286513));
#13188=CARTESIAN_POINT('',(3.5,14.8473002758614,247.086209595194));
#13189=CARTESIAN_POINT('',(3.5,14.8473002758614,253.771796440853));
#13190=CARTESIAN_POINT('',(-6.5,14.8473002758614,247.086209595194));
#13191=CARTESIAN_POINT('Origin',(-6.5,15.8473002758613,250.657383286513));
#13192=CARTESIAN_POINT('',(3.5,15.0089220887177,251.202472284128));
#13193=CARTESIAN_POINT('',(-6.5,15.0089220887177,251.202472284128));
#13194=CARTESIAN_POINT('Origin',(3.5,15.8473002758613,250.657383286513));
#13195=CARTESIAN_POINT('Origin',(-6.5,16.7024755322828,253.80725475462));
#13196=CARTESIAN_POINT('',(-16.5,15.0089220887177,251.202472284128));
#13197=CARTESIAN_POINT('',(-6.5,15.0089220887177,251.202472284128));
#13198=CARTESIAN_POINT('',(-16.5,16.7024755322828,253.80725475462));
#13199=CARTESIAN_POINT('',(-16.5,14.3945664389275,250.257558007404));
#13200=CARTESIAN_POINT('',(3.5,16.7024755322828,253.80725475462));
#13201=CARTESIAN_POINT('',(-6.5,16.7024755322828,253.80725475462));
#13202=CARTESIAN_POINT('',(3.5,17.3657865921442,254.827465263934));
#13203=CARTESIAN_POINT('Origin',(-6.5,15.8473002758613,250.657383286513));
#13204=CARTESIAN_POINT('',(-16.5,14.8473002758614,250.657383286513));
#13205=CARTESIAN_POINT('',(-6.5,14.8473002758614,250.657383286513));
#13206=CARTESIAN_POINT('Origin',(-16.5,15.8473002758613,250.657383286513));
#13207=CARTESIAN_POINT('Origin',(-6.5,14.8473002758614,250.657383286513));
#13208=CARTESIAN_POINT('',(-16.5,14.8473002758614,247.086209595194));
#13209=CARTESIAN_POINT('',(-6.5,14.8473002758614,247.086209595194));
#13210=CARTESIAN_POINT('',(-16.5,14.8473002758614,253.771796440853));
#13211=CARTESIAN_POINT('Origin',(-6.5,14.6473002758614,247.086209595194));
#13212=CARTESIAN_POINT('',(-16.5,14.6473002758614,246.886209595194));
#13213=CARTESIAN_POINT('',(-6.5,14.6473002758614,246.886209595194));
#13214=CARTESIAN_POINT('Origin',(-16.5,14.6473002758614,247.086209595194));
#13215=CARTESIAN_POINT('Origin',(-6.5,6.43177298256785,247.086209595194));
#13216=CARTESIAN_POINT('',(-15.5,6.43177298256785,247.086209595194));
#13217=CARTESIAN_POINT('Origin',(-6.5,6.43177298256785,247.086209595194));
#13218=CARTESIAN_POINT('',(-10.5506510928848,-1.60515589130626,247.086209595194));
#13219=CARTESIAN_POINT('Origin',(-6.5,6.43177298256785,247.086209595194));
#13220=CARTESIAN_POINT('',(-10.6406655616155,-1.7837543107257,246.886209595194));
#13221=CARTESIAN_POINT('Origin',(-10.6406655616155,-1.7837543107257,247.086209595194));
#13222=CARTESIAN_POINT('Origin',(-6.5,6.43177298256785,246.886209595194));
#13223=CARTESIAN_POINT('Origin',(-2.35933443838448,-1.7837543107257,247.086209595194));
#13224=CARTESIAN_POINT('',(-2.35933443838448,-1.9837543107257,247.086209595194));
#13225=CARTESIAN_POINT('',(-2.44934890711525,-1.60515589130627,247.086209595194));
#13226=CARTESIAN_POINT('Origin',(-2.35933443838448,-1.7837543107257,247.086209595194));
#13227=CARTESIAN_POINT('',(-2.35933443838448,-1.7837543107257,246.886209595194));
#13228=CARTESIAN_POINT('Origin',(-2.35933443838448,-1.7837543107257,247.086209595194));
#13229=CARTESIAN_POINT('Origin',(-2.35933443838448,-1.7837543107257,247.086209595194));
#13230=CARTESIAN_POINT('Origin',(-2.35933443838445,-1.78375431072568,256.886209595194));
#13231=CARTESIAN_POINT('',(-2.35933443838445,-1.98375431072569,250.657383286513));
#13232=CARTESIAN_POINT('',(-2.44934890711523,-1.60515589130626,250.657383286513));
#13233=CARTESIAN_POINT('Origin',(-2.35933443838445,-1.78375431072568,250.657383286513));
#13234=CARTESIAN_POINT('',(-2.44934890711523,-1.60515589130626,256.886209595194));
#13235=CARTESIAN_POINT('',(-2.35933443838445,-1.98375431072568,256.886209595194));
#13236=CARTESIAN_POINT('Ctrl Pts',(-2.35933443838447,-1.98375431072569,
250.657383286513));
#13237=CARTESIAN_POINT('Ctrl Pts',(-2.35933443838446,-1.98375431072569,
250.772822299168));
#13238=CARTESIAN_POINT('Ctrl Pts',(-2.46187926199705,-2.02731361034112,
250.995273610107));
#13239=CARTESIAN_POINT('Ctrl Pts',(-2.66151050029649,-2.10565390596992,
251.141377231877));
#13240=CARTESIAN_POINT('Ctrl Pts',(-2.7689470683364,-2.14537612358201,251.202472284128));
#13241=CARTESIAN_POINT('Ctrl Pts',(-2.4102819870235,-1.98375431072569,250.657383286513));
#13242=CARTESIAN_POINT('Ctrl Pts',(-2.41028198702349,-1.98375431072569,
250.761141960988));
#13243=CARTESIAN_POINT('Ctrl Pts',(-2.50259327156958,-2.01836361311809,
250.965068838285));
#13244=CARTESIAN_POINT('Ctrl Pts',(-2.69407745702402,-2.08894977673007,
251.110832462786));
#13245=CARTESIAN_POINT('Ctrl Pts',(-2.79833310653511,-2.12569665959276,
251.172204138164));
#13246=CARTESIAN_POINT('Ctrl Pts',(-2.51184443386601,-1.94270545541938,
250.657383286513));
#13247=CARTESIAN_POINT('Ctrl Pts',(-2.511844433866,-1.94270545541938,250.742595721283));
#13248=CARTESIAN_POINT('Ctrl Pts',(-2.58378619591607,-1.96368057545467,
250.91832476734));
#13249=CARTESIAN_POINT('Ctrl Pts',(-2.7590798598131,-2.02453104301038,251.06710566137));
#13250=CARTESIAN_POINT('Ctrl Pts',(-2.85696933307462,-2.05794641939893,
251.130326126116));
#13251=CARTESIAN_POINT('Ctrl Pts',(-2.57981436360185,-1.79296837898676,
250.657383286513));
#13252=CARTESIAN_POINT('Ctrl Pts',(-2.57981436360184,-1.79296837898676,
250.74435628427));
#13253=CARTESIAN_POINT('Ctrl Pts',(-2.64258917521035,-1.81562445015628,
250.925879430023));
#13254=CARTESIAN_POINT('Ctrl Pts',(-2.80949734511231,-1.8822863779169,251.084602122621));
#13255=CARTESIAN_POINT('Ctrl Pts',(-2.90391764800065,-1.91879256215878,
251.152000466197));
#13256=CARTESIAN_POINT('Ctrl Pts',(-2.53401156509197,-1.66390087931709,
250.657383286513));
#13257=CARTESIAN_POINT('Ctrl Pts',(-2.53401156509196,-1.66390087931709,
250.769730689184));
#13258=CARTESIAN_POINT('Ctrl Pts',(-2.61306596902394,-1.70195279380099,
250.993661548375));
#13259=CARTESIAN_POINT('Ctrl Pts',(-2.79160486243893,-1.78331601786504,
251.161662294744));
#13260=CARTESIAN_POINT('Ctrl Pts',(-2.89026067918543,-1.82587649606285,
251.232425097961));
#13261=CARTESIAN_POINT('Ctrl Pts',(-2.4720967862658,-1.61662093261596,250.657383286513));
#13262=CARTESIAN_POINT('Ctrl Pts',(-2.4720967862658,-1.61662093261596,250.789388896833));
#13263=CARTESIAN_POINT('Ctrl Pts',(-2.56697742498125,-1.66465600150291,
251.045597335));
#13264=CARTESIAN_POINT('Ctrl Pts',(-2.75789762139033,-1.75418178955874,
251.219068720891));
#13265=CARTESIAN_POINT('Ctrl Pts',(-2.86131674875401,-1.79988152535352,
251.291741549006));
#13266=CARTESIAN_POINT('Ctrl Pts',(-2.44934890711524,-1.60515589130627,
250.657383286513));
#13267=CARTESIAN_POINT('Ctrl Pts',(-2.44934890711524,-1.60515589130626,
250.795910101699));
#13268=CARTESIAN_POINT('Ctrl Pts',(-2.5496644954319,-1.65629072128959,251.062851674826));
#13269=CARTESIAN_POINT('Ctrl Pts',(-2.74495592420308,-1.74825541615818,
251.23817602095));
#13270=CARTESIAN_POINT('Ctrl Pts',(-2.85005691467691,-1.7948858455289,251.311490083651));
#13271=CARTESIAN_POINT('',(-2.7689470683364,-2.14537612358201,251.202472284128));
#13272=CARTESIAN_POINT('',(-2.85005691467691,-1.7948858455289,251.311490083651));
#13273=CARTESIAN_POINT('Origin',(-2.7689470683364,-1.97770048615327,251.311490083651));
#13274=CARTESIAN_POINT('Ctrl Pts',(-2.85005691467691,-1.7948858455289,251.311490083651));
#13275=CARTESIAN_POINT('Ctrl Pts',(-2.74495592420308,-1.74825541615818,
251.23817602095));
#13276=CARTESIAN_POINT('Ctrl Pts',(-2.5496644954319,-1.65629072128959,251.062851674826));
#13277=CARTESIAN_POINT('Ctrl Pts',(-2.44934890711524,-1.60515589130626,
250.795910101699));
#13278=CARTESIAN_POINT('Ctrl Pts',(-2.44934890711524,-1.60515589130627,
250.657383286513));
#13279=CARTESIAN_POINT('Ctrl Pts',(-2.35933443838447,-1.98375431072569,
250.657383286513));
#13280=CARTESIAN_POINT('Ctrl Pts',(-2.35933443838446,-1.98375431072569,
250.772822299168));
#13281=CARTESIAN_POINT('Ctrl Pts',(-2.46187926199705,-2.02731361034112,
250.995273610107));
#13282=CARTESIAN_POINT('Ctrl Pts',(-2.66151050029649,-2.10565390596992,
251.141377231877));
#13283=CARTESIAN_POINT('Ctrl Pts',(-2.7689470683364,-2.14537612358201,251.202472284128));
#13284=CARTESIAN_POINT('Ctrl Pts',(-2.7689470683364,-2.14537612358201,251.202472284128));
#13285=CARTESIAN_POINT('Ctrl Pts',(-3.77226840311965,-2.59052230561913,
251.887132680399));
#13286=CARTESIAN_POINT('Ctrl Pts',(-5.57837183813838,-3.0292444933001,252.561912604368));
#13287=CARTESIAN_POINT('Ctrl Pts',(-8.15338081673582,-2.87490004729592,
252.324521981181));
#13288=CARTESIAN_POINT('Ctrl Pts',(-9.56217204180809,-2.44214024494009,
251.658912548309));
#13289=CARTESIAN_POINT('Ctrl Pts',(-10.2310529316636,-2.14537612358201,
251.202472284128));
#13290=CARTESIAN_POINT('Ctrl Pts',(-2.79833310653511,-2.12569665959276,
251.172204138164));
#13291=CARTESIAN_POINT('Ctrl Pts',(-3.79672716582859,-2.5678363253453,251.852198827549));
#13292=CARTESIAN_POINT('Ctrl Pts',(-5.58802871625117,-3.00150512886098,
252.519153595767));
#13293=CARTESIAN_POINT('Ctrl Pts',(-8.13659337144744,-2.84912459574666,
252.284803763196));
#13294=CARTESIAN_POINT('Ctrl Pts',(-9.53607085393589,-2.42045643676112,
251.625533931087));
#13295=CARTESIAN_POINT('Ctrl Pts',(-10.2016668934649,-2.12569665959276,
251.172204138164));
#13296=CARTESIAN_POINT('Ctrl Pts',(-2.85696935144547,-2.05794617860782,
251.13032625575));
#13297=CARTESIAN_POINT('Ctrl Pts',(-3.84550834632558,-2.49248211993982,
251.802015209738));
#13298=CARTESIAN_POINT('Ctrl Pts',(-5.60737730602117,-2.91405769435918,
252.454604565079));
#13299=CARTESIAN_POINT('Ctrl Pts',(-8.10304493491812,-2.76633681628283,
252.225863919145));
#13300=CARTESIAN_POINT('Ctrl Pts',(-9.48400465196778,-2.34763680616248,
251.578118891742));
#13301=CARTESIAN_POINT('Ctrl Pts',(-10.1430306485545,-2.05794617860782,
251.13032625575));
#13302=CARTESIAN_POINT('Ctrl Pts',(-2.90391767111428,-1.91879244249013,
251.152000510131));
#13303=CARTESIAN_POINT('Ctrl Pts',(-3.88254920604482,-2.34506924067967,
251.82148239871));
#13304=CARTESIAN_POINT('Ctrl Pts',(-5.62105275595405,-2.75575651795704,
252.469871929561));
#13305=CARTESIAN_POINT('Ctrl Pts',(-8.07893705070351,-2.61209324920213,
252.242793964634));
#13306=CARTESIAN_POINT('Ctrl Pts',(-9.44366130559868,-2.2029769746165,251.598321769183));
#13307=CARTESIAN_POINT('Ctrl Pts',(-10.0960823288857,-1.91879244249013,
251.152000510131));
#13308=CARTESIAN_POINT('Ctrl Pts',(-2.89026069830919,-1.82587639593774,
251.232425135035));
#13309=CARTESIAN_POINT('Ctrl Pts',(-3.86765930897934,-2.2537442325047,251.90907507138));
#13310=CARTESIAN_POINT('Ctrl Pts',(-5.61370506773033,-2.66971313360356,
252.569860268798));
#13311=CARTESIAN_POINT('Ctrl Pts',(-8.09123862855148,-2.52386111525648,
252.33794267841));
#13312=CARTESIAN_POINT('Ctrl Pts',(-9.4581402279107,-2.11112162031572,251.683525092599));
#13313=CARTESIAN_POINT('Ctrl Pts',(-10.1097393016908,-1.82587639593775,
251.232425135035));
#13314=CARTESIAN_POINT('Ctrl Pts',(-2.86131674875401,-1.79988152535352,
251.291741549006));
#13315=CARTESIAN_POINT('Ctrl Pts',(-3.84154141667882,-2.23319023011266,
251.97440989295));
#13316=CARTESIAN_POINT('Ctrl Pts',(-5.60252881155338,-2.65875979334497,
252.645711029322));
#13317=CARTESIAN_POINT('Ctrl Pts',(-8.11031912498652,-2.50916768931843,
252.40968064353));
#13318=CARTESIAN_POINT('Ctrl Pts',(-9.48520013929611,-2.08875399519296,
251.746853778302));
#13319=CARTESIAN_POINT('Ctrl Pts',(-10.138683251246,-1.79988152535353,251.291741549006));
#13320=CARTESIAN_POINT('Ctrl Pts',(-2.85005691467691,-1.7948858455289,251.311490083651));
#13321=CARTESIAN_POINT('Ctrl Pts',(-3.83156691609531,-2.23035493665217,
251.996150479922));
#13322=CARTESIAN_POINT('Ctrl Pts',(-5.59840723296145,-2.65953968547052,
252.670930403891));
#13323=CARTESIAN_POINT('Ctrl Pts',(-8.11743775550243,-2.5085505535099,252.433539780704));
#13324=CARTESIAN_POINT('Ctrl Pts',(-9.49560308437748,-2.08519857294442,
251.767930347832));
#13325=CARTESIAN_POINT('Ctrl Pts',(-10.1499430853231,-1.79488584552891,
251.311490083651));
#13326=CARTESIAN_POINT('',(-10.2310529316636,-2.14537612358201,251.202472284128));
#13327=CARTESIAN_POINT('',(-10.1499430853231,-1.79488584552891,251.311490083651));
#13328=CARTESIAN_POINT('Origin',(-10.2310529316636,-1.97770048615328,251.311490083651));
#13329=CARTESIAN_POINT('Origin',(-6.5,6.43177298256785,238.377236865592));
#13330=CARTESIAN_POINT('Origin',(-6.5,6.26409734513912,238.268219066069));
#13331=CARTESIAN_POINT('Ctrl Pts',(-10.2310529316636,-2.14537612358201,
251.202472284128));
#13332=CARTESIAN_POINT('Ctrl Pts',(-10.3384971542717,-2.10565107586813,
251.141372879018));
#13333=CARTESIAN_POINT('Ctrl Pts',(-10.5381140246013,-2.02731718901882,
250.995305028042));
#13334=CARTESIAN_POINT('Ctrl Pts',(-10.6406655616155,-1.98375431072569,
250.772830523889));
#13335=CARTESIAN_POINT('Ctrl Pts',(-10.6406655616155,-1.98375431072569,
250.657383286513));
#13336=CARTESIAN_POINT('Ctrl Pts',(-10.2016668934649,-2.12569665959276,
251.172204138164));
#13337=CARTESIAN_POINT('Ctrl Pts',(-10.3059299709122,-2.08894715861293,
251.110828090218));
#13338=CARTESIAN_POINT('Ctrl Pts',(-10.4974012709103,-2.01836605599956,
250.965097544891));
#13339=CARTESIAN_POINT('Ctrl Pts',(-10.5897180129765,-1.98375431072569,
250.761149353516));
#13340=CARTESIAN_POINT('Ctrl Pts',(-10.5897180129765,-1.98375431072569,
250.657383286513));
#13341=CARTESIAN_POINT('Ctrl Pts',(-10.1430306485535,-2.05794617859384,
251.130326255758));
#13342=CARTESIAN_POINT('Ctrl Pts',(-10.2409270961782,-2.02452842144907,
251.067101286723));
#13343=CARTESIAN_POINT('Ctrl Pts',(-10.4162108293298,-1.96368091150233,
250.918349437673));
#13344=CARTESIAN_POINT('Ctrl Pts',(-10.4881555222276,-1.94270505090509,
250.742601792441));
#13345=CARTESIAN_POINT('Ctrl Pts',(-10.4881555222275,-1.94270505090509,
250.657383286512));
#13346=CARTESIAN_POINT('Ctrl Pts',(-10.0960823288844,-1.91879244248318,
251.152000510133));
#13347=CARTESIAN_POINT('Ctrl Pts',(-10.1905093589668,-1.88228365727328,
251.084597364605));
#13348=CARTESIAN_POINT('Ctrl Pts',(-10.3574089229965,-1.8156250085404,250.925904890041));
#13349=CARTESIAN_POINT('Ctrl Pts',(-10.4201855817356,-1.79296819025683,
250.744362480863));
#13350=CARTESIAN_POINT('Ctrl Pts',(-10.4201855817356,-1.79296819025684,
250.657383286513));
#13351=CARTESIAN_POINT('Ctrl Pts',(-10.1097393016897,-1.82587639593193,
251.232425135037));
#13352=CARTESIAN_POINT('Ctrl Pts',(-10.2084021473994,-1.78331288541385,
251.16165729016));
#13353=CARTESIAN_POINT('Ctrl Pts',(-10.3869300787649,-1.70195523407075,
250.993693094235));
#13354=CARTESIAN_POINT('Ctrl Pts',(-10.4659883891908,-1.66390072133625,
250.769738693635));
#13355=CARTESIAN_POINT('Ctrl Pts',(-10.4659883891907,-1.66390072133626,
250.657383286512));
#13356=CARTESIAN_POINT('Ctrl Pts',(-10.138683251246,-1.79988152535352,251.291741549006));
#13357=CARTESIAN_POINT('Ctrl Pts',(-10.242109746946,-1.75417853357476,251.219063543146));
#13358=CARTESIAN_POINT('Ctrl Pts',(-10.4330166775059,-1.66465981113938,
251.04563349778));
#13359=CARTESIAN_POINT('Ctrl Pts',(-10.5279032137342,-1.61662093261595,
250.789398301879));
#13360=CARTESIAN_POINT('Ctrl Pts',(-10.5279032137342,-1.61662093261596,
250.657383286513));
#13361=CARTESIAN_POINT('Ctrl Pts',(-10.1499430853231,-1.7948858455289,251.311490083651));
#13362=CARTESIAN_POINT('Ctrl Pts',(-10.2550515639615,-1.74825209386477,
251.238170797519));
#13363=CARTESIAN_POINT('Ctrl Pts',(-10.45032893711,-1.65629492234602,251.062889376348));
#13364=CARTESIAN_POINT('Ctrl Pts',(-10.5506510928848,-1.60515589130626,
250.795919971364));
#13365=CARTESIAN_POINT('Ctrl Pts',(-10.5506510928848,-1.60515589130627,
250.657383286513));
#13366=CARTESIAN_POINT('',(-10.6406655616155,-1.98375431072569,250.657383286513));
#13367=CARTESIAN_POINT('',(-10.5506510928848,-1.60515589130627,250.657383286513));
#13368=CARTESIAN_POINT('Origin',(-10.6406655616155,-1.78375431072569,250.657383286513));
#13369=CARTESIAN_POINT('Ctrl Pts',(-10.5506510928848,-1.60515589130627,
250.657383286513));
#13370=CARTESIAN_POINT('Ctrl Pts',(-10.5506510928848,-1.60515589130626,
250.795919971364));
#13371=CARTESIAN_POINT('Ctrl Pts',(-10.45032893711,-1.65629492234602,251.062889376348));
#13372=CARTESIAN_POINT('Ctrl Pts',(-10.2550515639615,-1.74825209386477,
251.238170797519));
#13373=CARTESIAN_POINT('Ctrl Pts',(-10.1499430853231,-1.7948858455289,251.311490083651));
#13374=CARTESIAN_POINT('Ctrl Pts',(-10.2310529316636,-2.14537612358201,
251.202472284128));
#13375=CARTESIAN_POINT('Ctrl Pts',(-10.3384971542717,-2.10565107586813,
251.141372879018));
#13376=CARTESIAN_POINT('Ctrl Pts',(-10.5381140246013,-2.02731718901882,
250.995305028042));
#13377=CARTESIAN_POINT('Ctrl Pts',(-10.6406655616155,-1.98375431072569,
250.772830523889));
#13378=CARTESIAN_POINT('Ctrl Pts',(-10.6406655616155,-1.98375431072569,
250.657383286513));
#13379=CARTESIAN_POINT('Origin',(-10.6406655616155,-1.78375431072568,256.886209595194));
#13380=CARTESIAN_POINT('',(-10.6406655616155,-1.9837543107257,247.086209595194));
#13381=CARTESIAN_POINT('Origin',(-10.6406655616155,-1.78375431072568,247.086209595194));
#13382=CARTESIAN_POINT('',(-10.5506510928848,-1.60515589130626,256.886209595194));
#13383=CARTESIAN_POINT('',(-10.6406655616155,-1.98375431072568,256.886209595194));
#13384=CARTESIAN_POINT('Origin',(-10.6406655616155,-1.7837543107257,247.086209595194));
#13385=CARTESIAN_POINT('Origin',(-10.6406655616155,-1.7837543107257,247.086209595194));
#13386=CARTESIAN_POINT('Origin',(-6.5,-1.9837543107257,246.886209595194));
#13387=CARTESIAN_POINT('',(-16.5,-1.98375431072569,250.657383286513));
#13388=CARTESIAN_POINT('',(-6.5,-1.98375431072569,250.657383286513));
#13389=CARTESIAN_POINT('',(-16.5,-1.9837543107257,247.086209595194));
#13390=CARTESIAN_POINT('',(-16.5,-1.98375431072569,251.886209595194));
#13391=CARTESIAN_POINT('',(-6.5,-1.9837543107257,247.086209595194));
#13392=CARTESIAN_POINT('Origin',(-6.5,-2.98375431072556,250.657383286513));
#13393=CARTESIAN_POINT('',(-16.5,-2.14537612358201,251.202472284128));
#13394=CARTESIAN_POINT('',(-6.5,-2.14537612358201,251.202472284128));
#13395=CARTESIAN_POINT('Origin',(-16.5,-2.98375431072556,250.657383286513));
#13396=CARTESIAN_POINT('Origin',(-6.5,-2.14537612358201,251.202472284128));
#13397=CARTESIAN_POINT('',(3.5,-2.14537612358201,251.202472284128));
#13398=CARTESIAN_POINT('',(-6.5,-2.14537612358201,251.202472284128));
#13399=CARTESIAN_POINT('',(3.5,-3.83892956714709,253.80725475462));
#13400=CARTESIAN_POINT('',(3.5,-0.684243752009264,248.955166772158));
#13401=CARTESIAN_POINT('',(-16.5,-3.83892956714709,253.80725475462));
#13402=CARTESIAN_POINT('',(-6.5,-3.83892956714709,253.80725475462));
#13403=CARTESIAN_POINT('',(-16.5,-3.65546390522595,253.525074028688));
#13404=CARTESIAN_POINT('Origin',(-6.5,-2.98375431072556,250.657383286513));
#13405=CARTESIAN_POINT('',(3.5,-1.98375431072569,250.657383286513));
#13406=CARTESIAN_POINT('',(-6.5,-1.98375431072569,250.657383286513));
#13407=CARTESIAN_POINT('Origin',(3.5,-2.98375431072556,250.657383286513));
#13408=CARTESIAN_POINT('Origin',(-6.5,-1.9837543107257,246.886209595194));
#13409=CARTESIAN_POINT('',(3.5,-1.9837543107257,247.086209595194));
#13410=CARTESIAN_POINT('',(-6.5,-1.9837543107257,247.086209595194));
#13411=CARTESIAN_POINT('',(3.5,-1.98375431072569,251.886209595194));
#13412=CARTESIAN_POINT('Origin',(-6.5,-1.7837543107257,247.086209595194));
#13413=CARTESIAN_POINT('',(3.5,-1.7837543107257,246.886209595194));
#13414=CARTESIAN_POINT('',(-6.5,-1.7837543107257,246.886209595194));
#13415=CARTESIAN_POINT('Origin',(3.5,-1.7837543107257,247.086209595194));
#13416=CARTESIAN_POINT('Origin',(-6.5,6.43177298256785,247.086209595194));
#13417=CARTESIAN_POINT('Origin',(-6.5,6.43177298256785,246.886209595194));
#13418=CARTESIAN_POINT('Origin',(-6.5,6.43177298256785,247.086209595194));
#13419=CARTESIAN_POINT('Origin',(-6.5,14.6473002758614,247.086209595194));
#13420=CARTESIAN_POINT('',(3.5,14.6473002758614,246.886209595194));
#13421=CARTESIAN_POINT('Origin',(3.5,14.6473002758614,247.086209595194));
#13422=CARTESIAN_POINT('',(-6.5,14.6473002758614,246.886209595194));
#13423=CARTESIAN_POINT('Ctrl Pts',(3.7,14.4473002758614,246.886209595194));
#13424=CARTESIAN_POINT('Ctrl Pts',(3.7,14.6473002758614,246.886209595194));
#13425=CARTESIAN_POINT('Ctrl Pts',(3.5,14.6473002758614,246.886209595194));
#13426=CARTESIAN_POINT('Ctrl Pts',(3.90000000000004,14.4473002758614,246.886209595194));
#13427=CARTESIAN_POINT('Ctrl Pts',(3.90000000000004,14.8473002758614,246.886209595194));
#13428=CARTESIAN_POINT('Ctrl Pts',(3.5,14.8473002758614,246.886209595194));
#13429=CARTESIAN_POINT('Ctrl Pts',(3.9,14.4473002758614,247.086209595194));
#13430=CARTESIAN_POINT('Ctrl Pts',(3.9,14.8473002758614,247.086209595194));
#13431=CARTESIAN_POINT('Ctrl Pts',(3.5,14.8473002758614,247.086209595194));
#13432=CARTESIAN_POINT('',(3.9,14.4473002758614,247.086209595194));
#13433=CARTESIAN_POINT('',(3.7,14.4473002758614,246.886209595194));
#13434=CARTESIAN_POINT('Origin',(3.7,14.4473002758614,247.086209595194));
#13435=CARTESIAN_POINT('Origin',(3.5,14.4473002758614,246.886209595194));
#13436=CARTESIAN_POINT('Origin',(3.5,14.4473002758614,247.086209595194));
#13437=CARTESIAN_POINT('Origin',(3.7,11.4317729825679,247.086209595194));
#13438=CARTESIAN_POINT('',(3.9,-1.5837543107257,247.086209595194));
#13439=CARTESIAN_POINT('',(3.7,-1.5837543107257,246.886209595194));
#13440=CARTESIAN_POINT('Origin',(3.7,-1.5837543107257,247.086209595194));
#13441=CARTESIAN_POINT('',(3.7,11.4317729825679,246.886209595194));
#13442=CARTESIAN_POINT('',(3.9,11.4317729825679,247.086209595194));
#13443=CARTESIAN_POINT('Ctrl Pts',(3.5,-1.7837543107257,246.886209595194));
#13444=CARTESIAN_POINT('Ctrl Pts',(3.7,-1.7837543107257,246.886209595194));
#13445=CARTESIAN_POINT('Ctrl Pts',(3.7,-1.5837543107257,246.886209595194));
#13446=CARTESIAN_POINT('Ctrl Pts',(3.5,-1.9837543107257,246.886209595194));
#13447=CARTESIAN_POINT('Ctrl Pts',(3.9,-1.9837543107257,246.886209595194));
#13448=CARTESIAN_POINT('Ctrl Pts',(3.9,-1.5837543107257,246.886209595194));
#13449=CARTESIAN_POINT('Ctrl Pts',(3.5,-1.9837543107257,247.086209595194));
#13450=CARTESIAN_POINT('Ctrl Pts',(3.9,-1.9837543107257,247.086209595194));
#13451=CARTESIAN_POINT('Ctrl Pts',(3.9,-1.5837543107257,247.086209595194));
#13452=CARTESIAN_POINT('Origin',(3.5,-1.5837543107257,246.886209595194));
#13453=CARTESIAN_POINT('Origin',(3.5,-1.5837543107257,247.086209595194));
#13454=CARTESIAN_POINT('Origin',(3.5,14.4473002758614,253.771796440853));
#13455=CARTESIAN_POINT('',(3.9,14.4473002758614,250.657383286513));
#13456=CARTESIAN_POINT('Origin',(3.5,14.4473002758614,250.657383286513));
#13457=CARTESIAN_POINT('',(3.9,14.4473002758614,253.771796440853));
#13458=CARTESIAN_POINT('Origin',(-6.5,6.43177298256785,256.886209595194));
#13459=CARTESIAN_POINT('',(-15.5,6.43177298256785,256.886209595194));
#13460=CARTESIAN_POINT('Origin',(-6.5,6.43177298256785,246.886209595194));
#13461=CARTESIAN_POINT('Origin',(-6.5,-1.7837543107257,247.086209595194));
#13462=CARTESIAN_POINT('',(-16.5,-1.7837543107257,246.886209595194));
#13463=CARTESIAN_POINT('Origin',(-16.5,-1.7837543107257,247.086209595194));
#13464=CARTESIAN_POINT('',(-6.5,-1.7837543107257,246.886209595194));
#13465=CARTESIAN_POINT('Ctrl Pts',(-16.7,-1.5837543107257,246.886209595194));
#13466=CARTESIAN_POINT('Ctrl Pts',(-16.7,-1.7837543107257,246.886209595194));
#13467=CARTESIAN_POINT('Ctrl Pts',(-16.5,-1.7837543107257,246.886209595194));
#13468=CARTESIAN_POINT('Ctrl Pts',(-16.9,-1.5837543107257,246.886209595194));
#13469=CARTESIAN_POINT('Ctrl Pts',(-16.9,-1.9837543107257,246.886209595194));
#13470=CARTESIAN_POINT('Ctrl Pts',(-16.5,-1.9837543107257,246.886209595194));
#13471=CARTESIAN_POINT('Ctrl Pts',(-16.9,-1.5837543107257,247.086209595194));
#13472=CARTESIAN_POINT('Ctrl Pts',(-16.9,-1.9837543107257,247.086209595194));
#13473=CARTESIAN_POINT('Ctrl Pts',(-16.5,-1.9837543107257,247.086209595194));
#13474=CARTESIAN_POINT('',(-16.9,-1.5837543107257,247.086209595194));
#13475=CARTESIAN_POINT('',(-16.7,-1.5837543107257,246.886209595194));
#13476=CARTESIAN_POINT('Origin',(-16.7,-1.5837543107257,247.086209595194));
#13477=CARTESIAN_POINT('Origin',(-16.5,-1.5837543107257,246.886209595194));
#13478=CARTESIAN_POINT('Origin',(-16.5,-1.5837543107257,247.086209595194));
#13479=CARTESIAN_POINT('Origin',(-16.7,1.43177298256785,247.086209595194));
#13480=CARTESIAN_POINT('',(-16.9,14.4473002758614,247.086209595194));
#13481=CARTESIAN_POINT('',(-16.7,14.4473002758614,246.886209595194));
#13482=CARTESIAN_POINT('Origin',(-16.7,14.4473002758614,247.086209595194));
#13483=CARTESIAN_POINT('',(-16.7,1.43177298256785,246.886209595194));
#13484=CARTESIAN_POINT('',(-16.9,1.43177298256785,247.086209595194));
#13485=CARTESIAN_POINT('Ctrl Pts',(-16.5,14.6473002758614,246.886209595194));
#13486=CARTESIAN_POINT('Ctrl Pts',(-16.7,14.6473002758614,246.886209595194));
#13487=CARTESIAN_POINT('Ctrl Pts',(-16.7,14.4473002758614,246.886209595194));
#13488=CARTESIAN_POINT('Ctrl Pts',(-16.5,14.8473002758614,246.886209595194));
#13489=CARTESIAN_POINT('Ctrl Pts',(-16.9,14.8473002758614,246.886209595194));
#13490=CARTESIAN_POINT('Ctrl Pts',(-16.9,14.4473002758614,246.886209595194));
#13491=CARTESIAN_POINT('Ctrl Pts',(-16.5,14.8473002758614,247.086209595194));
#13492=CARTESIAN_POINT('Ctrl Pts',(-16.9,14.8473002758614,247.086209595194));
#13493=CARTESIAN_POINT('Ctrl Pts',(-16.9,14.4473002758614,247.086209595194));
#13494=CARTESIAN_POINT('Origin',(-16.5,14.4473002758614,246.886209595194));
#13495=CARTESIAN_POINT('Origin',(-16.5,14.4473002758614,247.086209595194));
#13496=CARTESIAN_POINT('Origin',(-16.5,-1.58375431072569,251.886209595194));
#13497=CARTESIAN_POINT('',(-16.9,-1.58375431072569,250.657383286513));
#13498=CARTESIAN_POINT('Origin',(-16.5,-1.58375431072569,250.657383286513));
#13499=CARTESIAN_POINT('',(-16.9,-1.58375431072569,251.886209595194));
#13500=CARTESIAN_POINT('Origin',(-6.5,6.43177298256785,246.886209595194));
#13501=CARTESIAN_POINT('Origin',(3.5,-0.348892477151795,249.173202371204));
#13502=CARTESIAN_POINT('',(3.9,-3.50357829228962,254.025290353666));
#13503=CARTESIAN_POINT('Origin',(3.5,-3.50357829228962,254.025290353666));
#13504=CARTESIAN_POINT('',(3.9,-1.81002484872454,251.420507883174));
#13505=CARTESIAN_POINT('Origin',(3.5,-1.81002484872454,251.420507883174));
#13506=CARTESIAN_POINT('',(3.9,-0.348892477151795,249.173202371204));
#13507=CARTESIAN_POINT('Origin',(3.5,-2.98375431072556,250.657383286513));
#13508=CARTESIAN_POINT('',(3.9,-1.58375431072569,250.657383286513));
#13509=CARTESIAN_POINT('Origin',(3.5,-1.58375431072569,250.657383286513));
#13510=CARTESIAN_POINT('Origin',(3.9,-2.98375431072556,250.657383286513));
#13511=CARTESIAN_POINT('Origin',(3.5,-1.58375431072569,251.886209595194));
#13512=CARTESIAN_POINT('',(3.9,-1.58375431072569,251.886209595194));
#13513=CARTESIAN_POINT('Ctrl Pts',(3.5,-3.96822701743216,254.243325952712));
#13514=CARTESIAN_POINT('Ctrl Pts',(3.5,-3.96822701743216,254.006121659742));
#13515=CARTESIAN_POINT('Ctrl Pts',(3.5,-3.83892956714706,253.80725475462));
#13516=CARTESIAN_POINT('Ctrl Pts',(3.90000000000001,-3.96822701743216,254.243325952712));
#13517=CARTESIAN_POINT('Ctrl Pts',(3.90000000000001,-3.96822701743216,254.006121659742));
#13518=CARTESIAN_POINT('Ctrl Pts',(3.90000000000001,-3.83892956714706,253.80725475462));
#13519=CARTESIAN_POINT('Ctrl Pts',(3.9,-3.56822701743216,254.243325952712));
#13520=CARTESIAN_POINT('Ctrl Pts',(3.9,-3.56822701743216,254.124723806227));
#13521=CARTESIAN_POINT('Ctrl Pts',(3.9,-3.50357829228961,254.025290353666));
#13522=CARTESIAN_POINT('',(3.9,-3.56822701743215,254.243325952712));
#13523=CARTESIAN_POINT('',(3.5,-3.96822701743215,254.243325952712));
#13524=CARTESIAN_POINT('Origin',(3.5,-3.56822701743216,254.243325952712));
#13525=CARTESIAN_POINT('Origin',(3.5,-3.1682270174321,254.243325952712));
#13526=CARTESIAN_POINT('Origin',(3.9,-3.1682270174321,254.243325952712));
#13527=CARTESIAN_POINT('Origin',(3.9,16.4317729825679,256.886209595194));
#13528=CARTESIAN_POINT('',(3.9,14.6735708138602,251.420507883175));
#13529=CARTESIAN_POINT('Origin',(3.9,15.8473002758613,250.657383286513));
#13530=CARTESIAN_POINT('',(3.9,16.3671242574253,254.025290353666));
#13531=CARTESIAN_POINT('',(3.9,17.0304353172867,255.04550086298));
#13532=CARTESIAN_POINT('',(3.9,16.4317729825679,254.243325952712));
#13533=CARTESIAN_POINT('Origin',(3.9,16.0317729825678,254.243325952712));
#13534=CARTESIAN_POINT('',(3.9,16.4317729825679,256.886209595194));
#13535=CARTESIAN_POINT('',(3.9,16.4317729825679,256.886209595194));
#13536=CARTESIAN_POINT('',(3.9,-3.56822701743215,256.886209595194));
#13537=CARTESIAN_POINT('',(3.9,11.4317729825679,256.886209595194));
#13538=CARTESIAN_POINT('',(3.9,-3.56822701743215,256.886209595194));
#13539=CARTESIAN_POINT('',(3.9,4.64187227009995,247.547898263196));
#13540=CARTESIAN_POINT('',(3.9,8.22167369503577,247.547898263196));
#13541=CARTESIAN_POINT('Origin',(3.9,6.43177298256785,249.937669285906));
#13542=CARTESIAN_POINT('',(3.9,10.5368226263339,247.547898263195));
#13543=CARTESIAN_POINT('Origin',(3.5,15.8473002758613,250.657383286513));
#13544=CARTESIAN_POINT('Origin',(3.5,14.6735708138602,251.420507883175));
#13545=CARTESIAN_POINT('Origin',(3.5,17.0304353172867,255.04550086298));
#13546=CARTESIAN_POINT('Origin',(3.5,16.3671242574253,254.025290353666));
#13547=CARTESIAN_POINT('Ctrl Pts',(3.5,16.7024755322828,253.80725475462));
#13548=CARTESIAN_POINT('Ctrl Pts',(3.5,16.8317729825679,254.006121659742));
#13549=CARTESIAN_POINT('Ctrl Pts',(3.5,16.8317729825679,254.243325952712));
#13550=CARTESIAN_POINT('Ctrl Pts',(3.9,16.7024755322828,253.80725475462));
#13551=CARTESIAN_POINT('Ctrl Pts',(3.9,16.8317729825679,254.006121659742));
#13552=CARTESIAN_POINT('Ctrl Pts',(3.9,16.8317729825679,254.243325952712));
#13553=CARTESIAN_POINT('Ctrl Pts',(3.9,16.3671242574253,254.025290353666));
#13554=CARTESIAN_POINT('Ctrl Pts',(3.9,16.4317729825679,254.124723806227));
#13555=CARTESIAN_POINT('Ctrl Pts',(3.9,16.4317729825679,254.243325952712));
#13556=CARTESIAN_POINT('',(3.5,16.8317729825679,254.243325952712));
#13557=CARTESIAN_POINT('Origin',(3.5,16.4317729825679,254.243325952712));
#13558=CARTESIAN_POINT('Origin',(3.5,16.0317729825678,254.243325952712));
#13559=CARTESIAN_POINT('Origin',(-16.5,14.05921516407,250.47559360645));
#13560=CARTESIAN_POINT('',(-16.9,16.3671242574253,254.025290353666));
#13561=CARTESIAN_POINT('Origin',(-16.5,16.3671242574253,254.025290353666));
#13562=CARTESIAN_POINT('',(-16.9,14.6735708138602,251.420507883174));
#13563=CARTESIAN_POINT('Origin',(-16.5,14.6735708138602,251.420507883174));
#13564=CARTESIAN_POINT('',(-16.9,14.05921516407,250.47559360645));
#13565=CARTESIAN_POINT('Origin',(-16.5,15.8473002758613,250.657383286513));
#13566=CARTESIAN_POINT('',(-16.9,14.4473002758614,250.657383286513));
#13567=CARTESIAN_POINT('Origin',(-16.5,14.4473002758614,250.657383286513));
#13568=CARTESIAN_POINT('Origin',(-16.9,15.8473002758613,250.657383286513));
#13569=CARTESIAN_POINT('Origin',(-16.5,14.4473002758614,253.771796440853));
#13570=CARTESIAN_POINT('',(-16.9,14.4473002758614,253.771796440853));
#13571=CARTESIAN_POINT('Ctrl Pts',(-16.5,16.8317729825679,254.243325952712));
#13572=CARTESIAN_POINT('Ctrl Pts',(-16.5,16.8317729825679,254.006121659742));
#13573=CARTESIAN_POINT('Ctrl Pts',(-16.5,16.7024755322828,253.80725475462));
#13574=CARTESIAN_POINT('Ctrl Pts',(-16.9,16.8317729825679,254.243325952712));
#13575=CARTESIAN_POINT('Ctrl Pts',(-16.9,16.8317729825679,254.006121659742));
#13576=CARTESIAN_POINT('Ctrl Pts',(-16.9,16.7024755322828,253.80725475462));
#13577=CARTESIAN_POINT('Ctrl Pts',(-16.9,16.4317729825679,254.243325952712));
#13578=CARTESIAN_POINT('Ctrl Pts',(-16.9,16.4317729825679,254.124723806227));
#13579=CARTESIAN_POINT('Ctrl Pts',(-16.9,16.3671242574253,254.025290353666));
#13580=CARTESIAN_POINT('',(-16.9,16.4317729825678,254.243325952712));
#13581=CARTESIAN_POINT('',(-16.5,16.8317729825679,254.243325952712));
#13582=CARTESIAN_POINT('Origin',(-16.5,16.4317729825679,254.243325952712));
#13583=CARTESIAN_POINT('Origin',(-16.5,16.0317729825678,254.243325952712));
#13584=CARTESIAN_POINT('Origin',(-16.9,16.0317729825678,254.243325952712));
#13585=CARTESIAN_POINT('Origin',(-16.9,-3.56822701743215,256.886209595194));
#13586=CARTESIAN_POINT('',(-16.9,-1.81002484872455,251.420507883175));
#13587=CARTESIAN_POINT('Origin',(-16.9,-2.98375431072556,250.657383286513));
#13588=CARTESIAN_POINT('',(-16.9,-3.50357829228962,254.025290353666));
#13589=CARTESIAN_POINT('',(-16.9,-3.32011263036848,253.743109627734));
#13590=CARTESIAN_POINT('',(-16.9,-3.56822701743215,254.243325952712));
#13591=CARTESIAN_POINT('Origin',(-16.9,-3.1682270174321,254.243325952712));
#13592=CARTESIAN_POINT('',(-16.9,-3.56822701743215,256.886209595194));
#13593=CARTESIAN_POINT('',(-16.9,-3.56822701743215,256.886209595194));
#13594=CARTESIAN_POINT('',(-16.9,16.4317729825678,256.886209595194));
#13595=CARTESIAN_POINT('',(-16.9,1.43177298256785,256.886209595194));
#13596=CARTESIAN_POINT('',(-16.9,16.4317729825678,256.886209595194));
#13597=CARTESIAN_POINT('',(-16.9,4.64187227009995,247.547898263196));
#13598=CARTESIAN_POINT('',(-16.9,8.22167369503577,247.547898263196));
#13599=CARTESIAN_POINT('',(-16.9,0.536822626333899,247.547898263195));
#13600=CARTESIAN_POINT('Origin',(-16.9,6.43177298256785,249.937669285906));
#13601=CARTESIAN_POINT('Origin',(-16.5,-2.98375431072556,250.657383286513));
#13602=CARTESIAN_POINT('Origin',(-16.5,-1.81002484872455,251.420507883175));
#13603=CARTESIAN_POINT('Origin',(-16.5,-3.32011263036848,253.743109627734));
#13604=CARTESIAN_POINT('Origin',(-16.5,-3.50357829228962,254.025290353666));
#13605=CARTESIAN_POINT('Ctrl Pts',(-16.5,-3.83892956714706,253.80725475462));
#13606=CARTESIAN_POINT('Ctrl Pts',(-16.5,-3.96822701743216,254.006121659742));
#13607=CARTESIAN_POINT('Ctrl Pts',(-16.5,-3.96822701743216,254.243325952712));
#13608=CARTESIAN_POINT('Ctrl Pts',(-16.9,-3.83892956714706,253.80725475462));
#13609=CARTESIAN_POINT('Ctrl Pts',(-16.9,-3.96822701743216,254.006121659742));
#13610=CARTESIAN_POINT('Ctrl Pts',(-16.9,-3.96822701743216,254.243325952712));
#13611=CARTESIAN_POINT('Ctrl Pts',(-16.9,-3.50357829228961,254.025290353666));
#13612=CARTESIAN_POINT('Ctrl Pts',(-16.9,-3.56822701743216,254.124723806227));
#13613=CARTESIAN_POINT('Ctrl Pts',(-16.9,-3.56822701743216,254.243325952712));
#13614=CARTESIAN_POINT('',(-16.5,-3.96822701743215,254.243325952712));
#13615=CARTESIAN_POINT('Origin',(-16.5,-3.56822701743216,254.243325952712));
#13616=CARTESIAN_POINT('Origin',(-16.5,-3.1682270174321,254.243325952712));
#13617=CARTESIAN_POINT('Origin',(-6.5,16.0317729825678,254.243325952712));
#13618=CARTESIAN_POINT('',(-6.5,16.8317729825679,254.243325952712));
#13619=CARTESIAN_POINT('Origin',(-6.5,-3.1682270174321,254.243325952712));
#13620=CARTESIAN_POINT('',(-6.5,-3.96822701743215,254.243325952712));
#13621=CARTESIAN_POINT('Origin',(-16.5,16.8317729825679,256.886209595194));
#13622=CARTESIAN_POINT('',(-16.5,16.8317729825679,256.886209595194));
#13623=CARTESIAN_POINT('',(-16.5,16.8317729825679,256.886209595194));
#13624=CARTESIAN_POINT('',(3.5,16.8317729825679,256.886209595194));
#13625=CARTESIAN_POINT('',(-11.5,16.8317729825679,256.886209595194));
#13626=CARTESIAN_POINT('',(3.5,16.8317729825679,256.886209595194));
#13627=CARTESIAN_POINT('Origin',(3.5,-3.96822701743215,256.886209595194));
#13628=CARTESIAN_POINT('',(3.5,-3.96822701743215,256.886209595194));
#13629=CARTESIAN_POINT('',(3.5,-3.96822701743215,256.886209595194));
#13630=CARTESIAN_POINT('',(-16.5,-3.96822701743215,256.886209595194));
#13631=CARTESIAN_POINT('',(-1.5,-3.96822701743215,256.886209595194));
#13632=CARTESIAN_POINT('',(-16.5,-3.96822701743215,256.886209595194));
#13633=CARTESIAN_POINT('Origin',(-6.5,6.43177298256785,249.937669285906));
#13634=CARTESIAN_POINT('',(5.5,4.64187227009995,247.547898263196));
#13635=CARTESIAN_POINT('',(-6.5,4.64187227009995,247.547898263196));
#13636=CARTESIAN_POINT('',(5.5,8.22167369503577,247.547898263196));
#13637=CARTESIAN_POINT('Origin',(5.5,6.43177298256785,249.937669285906));
#13638=CARTESIAN_POINT('',(-6.5,8.22167369503577,247.547898263196));
#13639=CARTESIAN_POINT('Origin',(-6.5,4.64187227009995,247.547898263196));
#13640=CARTESIAN_POINT('',(5.5,8.22167369503577,247.547898263196));
#13641=CARTESIAN_POINT('Origin',(5.5,6.43177298256785,250.235662713169));
#13642=CARTESIAN_POINT('Origin',(-6.5,4.64187227009995,247.547898263196));
#13643=CARTESIAN_POINT('',(-18.5,4.64187227009995,247.547898263196));
#13644=CARTESIAN_POINT('',(-6.5,4.64187227009995,247.547898263196));
#13645=CARTESIAN_POINT('',(-18.5,8.22167369503577,247.547898263196));
#13646=CARTESIAN_POINT('',(-18.5,8.22167369503577,247.547898263196));
#13647=CARTESIAN_POINT('',(-6.5,8.22167369503577,247.547898263196));
#13648=CARTESIAN_POINT('Origin',(-18.5,6.43177298256785,250.235662713169));
#13649=CARTESIAN_POINT('Origin',(-18.5,6.43177298256785,249.937669285906));
#13650=CARTESIAN_POINT('Origin',(-6.5,6.43177298256785,249.937669285906));
#13651=CARTESIAN_POINT('Origin',(-16.5,16.4317729825679,256.886209595194));
#13652=CARTESIAN_POINT('Origin',(-16.5,16.4317729825679,256.886209595194));
#13653=CARTESIAN_POINT('Origin',(-16.5,-3.56822701743215,256.886209595194));
#13654=CARTESIAN_POINT('Origin',(-16.5,-3.56822701743215,256.886209595194));
#13655=CARTESIAN_POINT('Origin',(3.5,-3.56822701743215,256.886209595194));
#13656=CARTESIAN_POINT('Origin',(3.5,-3.56822701743215,256.886209595194));
#13657=CARTESIAN_POINT('Origin',(3.5,16.4317729825678,256.886209595194));
#13658=CARTESIAN_POINT('Origin',(3.5,16.4317729825678,256.886209595194));
#13659=CARTESIAN_POINT('Origin',(-16.5,-3.56822701743215,256.886209595194));
#13660=CARTESIAN_POINT('',(-18.5,-3.56822701743215,256.886209595194));
#13661=CARTESIAN_POINT('',(-18.5,-3.56822701743215,256.886209595194));
#13662=CARTESIAN_POINT('Origin',(-16.5,-3.56822701743215,256.886209595194));
#13663=CARTESIAN_POINT('Origin',(-18.5,16.4317729825679,256.886209595194));
#13664=CARTESIAN_POINT('',(-18.5,16.4317729825679,256.886209595194));
#13665=CARTESIAN_POINT('',(-18.5,16.4317729825679,256.886209595194));
#13666=CARTESIAN_POINT('',(-18.5,16.4317729825679,256.886209595194));
#13667=CARTESIAN_POINT('Origin',(-16.5,16.4317729825679,256.886209595194));
#13668=CARTESIAN_POINT('',(-16.5,18.4317729825679,256.886209595194));
#13669=CARTESIAN_POINT('',(-16.5,18.4317729825679,256.886209595194));
#13670=CARTESIAN_POINT('Origin',(-16.5,16.4317729825679,256.886209595194));
#13671=CARTESIAN_POINT('Origin',(3.5,18.4317729825679,256.886209595194));
#13672=CARTESIAN_POINT('',(3.5,18.4317729825679,256.886209595194));
#13673=CARTESIAN_POINT('Origin',(-6.5,6.43177298256785,256.886209595194));
#17019=UNCERTAINTY_MEASURE_WITH_UNIT(LENGTH_MEASURE(0.01),#17043,
'DISTANCE_ACCURACY_VALUE',
'Maximum model space distance between geometric entities at asserted c
onnectivities');
#17028=UNCERTAINTY_MEASURE_WITH_UNIT(LENGTH_MEASURE(0.01),#17043,
'DISTANCE_ACCURACY_VALUE',
'Maximum model space distance between geometric entities at asserted c
onnectivities');
#17033=(
GEOMETRIC_REPRESENTATION_CONTEXT(3)
GLOBAL_UNCERTAINTY_ASSIGNED_CONTEXT((#17019))
GLOBAL_UNIT_ASSIGNED_CONTEXT((#17043,#17045,#17046))
REPRESENTATION_CONTEXT('','3D')
);
#17042=(
GEOMETRIC_REPRESENTATION_CONTEXT(3)
GLOBAL_UNCERTAINTY_ASSIGNED_CONTEXT((#17028))
GLOBAL_UNIT_ASSIGNED_CONTEXT((#17043,#17045,#17046))
REPRESENTATION_CONTEXT('','3D')
);
#17043=(
LENGTH_UNIT()
NAMED_UNIT(*)
SI_UNIT(.MILLI.,.METRE.)
);
#17045=(
NAMED_UNIT(*)
PLANE_ANGLE_UNIT()
SI_UNIT($,.RADIAN.)
);
#17046=(
NAMED_UNIT(*)
SI_UNIT($,.STERADIAN.)
SOLID_ANGLE_UNIT()
);
#17051=SHAPE_DEFINITION_REPRESENTATION(#17064,#17089);
#17064=PRODUCT_DEFINITION_SHAPE('',$,#17103);
#17089=SHAPE_REPRESENTATION('',(#8648),#17033);
#17098=PRODUCT_DEFINITION_CONTEXT('part definition',#17139,'design');
#17103=PRODUCT_DEFINITION('GUIDE','GUIDE',#17116,#17098);
#17116=PRODUCT_DEFINITION_FORMATION('',$,#17145);
#17139=APPLICATION_CONTEXT(
'Core Data for Automotive Mechanical Design Process');
#17140=PRODUCT_CONTEXT('part definition',#17139,'mechanical');
#17145=PRODUCT('GUIDE','GUIDE',$,(#17140));
#17154=PRESENTATION_STYLE_ASSIGNMENT((#17155));
#17155=SURFACE_STYLE_USAGE(.BOTH.,#17156);
#17156=SURFACE_SIDE_STYLE('',(#17157));
#17157=SURFACE_STYLE_FILL_AREA(#17158);
#17158=FILL_AREA_STYLE('Steel - Satin',(#17159));
#17159=FILL_AREA_STYLE_COLOUR('Steel - Satin',#17160);
#17160=COLOUR_RGB('Steel - Satin', 0.09019608, 0.27058824, 0.51372549);
ENDSEC;
END-ISO-10303-21;
